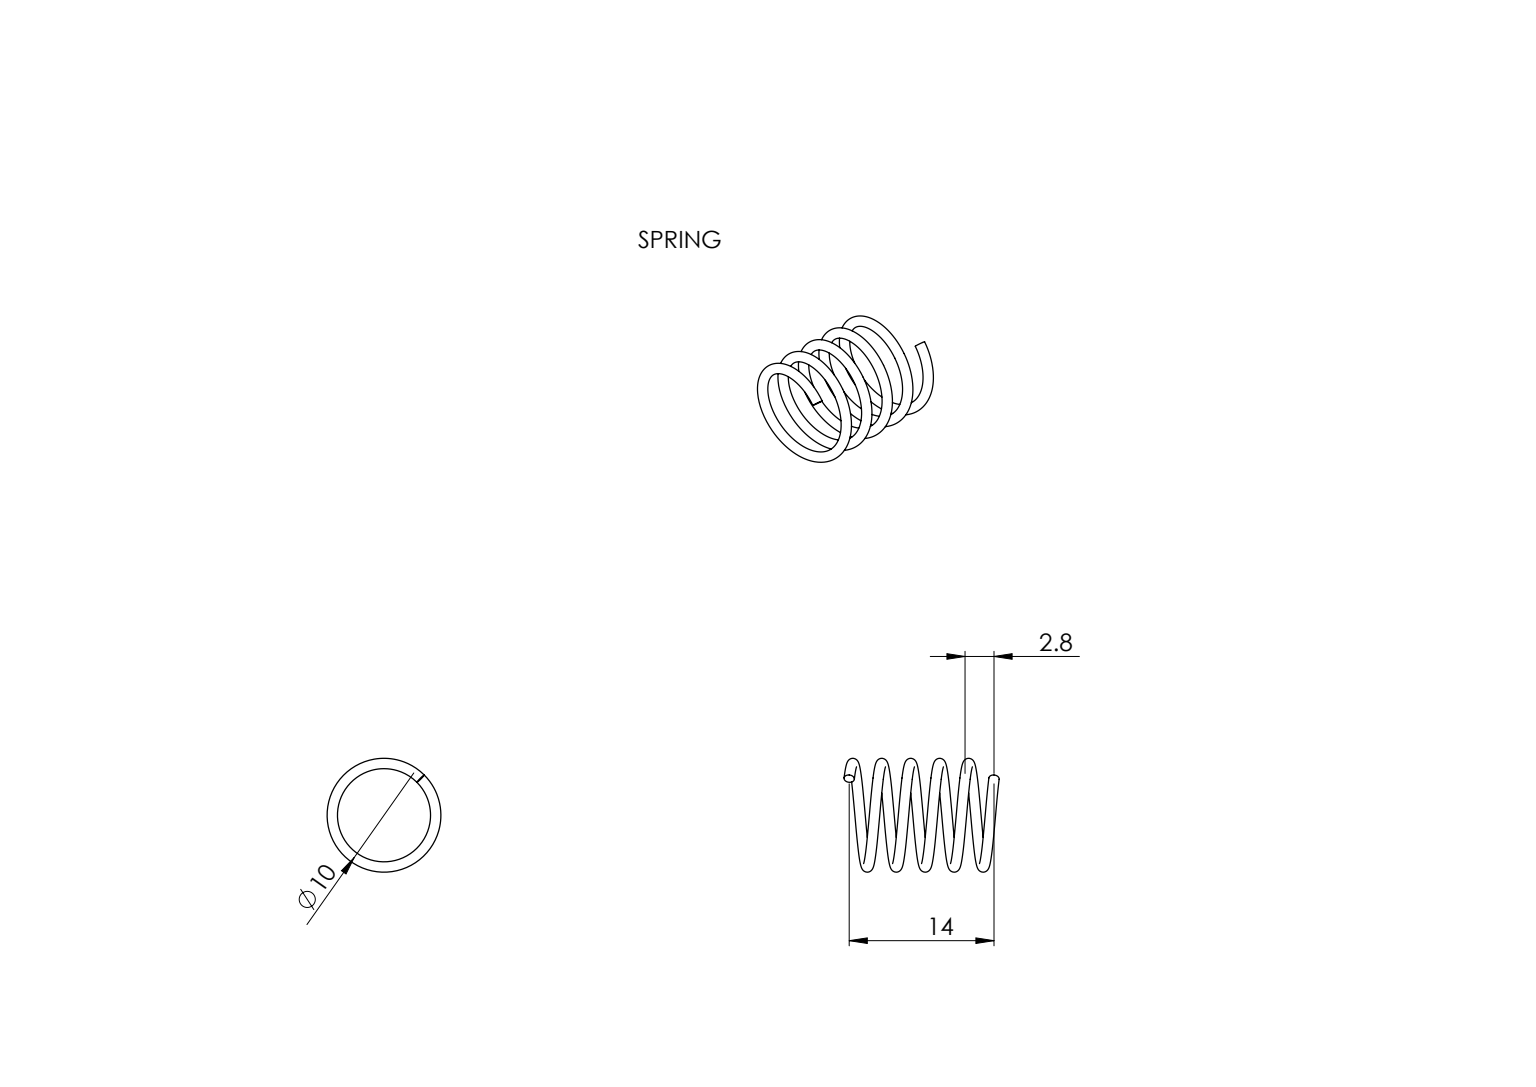
ISO-10303-21;
HEADER;
FILE_DESCRIPTION (('STEP AP214'),
    '1' );
FILE_NAME ('spring.step',
    '2026-10-03T18:28:46',
    ( '' ),
    ( '' ),
    'SwSTEP 2.0',
    'SolidWorks 2026',
    '' );
FILE_SCHEMA (( 'AUTOMOTIVE_DESIGN' ));
ENDSEC;

DATA;
#9=CARTESIAN_POINT ( 'NONE',  ( -2.231261971483764484, -4.173491630687871101, 3.063948283277976081 ) ) ;
#10=ORIENTED_EDGE ( 'NONE', *, *, #5513, .T. ) ;
#14=CARTESIAN_POINT ( 'NONE',  ( 4.089228379062037178, -4.089228379062022967, 0.6999999999999997335 ) ) ;
#18=CARTESIAN_POINT ( 'NONE',  ( 0.9046671180729953798, -5.711843387010016926, 0.9799999999999997602 ) ) ;
#30=CARTESIAN_POINT ( 'NONE',  ( 1.963858260114715870, -4.049832306626327316, 5.443948283277975975 ) ) ;
#40=CARTESIAN_POINT ( 'NONE',  ( 0.7401821875142697849, -4.673326407553650697, 3.779999999999998916 ) ) ;
#43=CARTESIAN_POINT ( 'NONE',  ( -0.9968613283357868893, 5.697241258616382531, 14.57605171672202538 ) ) ;
#49=CARTESIAN_POINT ( 'NONE',  ( 5.432285873273257515, 0.8603895577212793411, 8.679999999999997939 ) ) ;
#51=CARTESIAN_POINT ( 'NONE',  ( -3.889087296526005044, -3.889087296526019255, 1.399999999999999689 ) ) ;
#64=CARTESIAN_POINT ( 'NONE',  ( 3.244753828200538148, 3.119207202478391672, -0.9960517167220231949 ) ) ;
#67=CARTESIAN_POINT ( 'NONE',  ( -0.8603895577212598011, -5.432285873273260179, 6.719999999999999751 ) ) ;
#76=CARTESIAN_POINT ( 'NONE',  ( 4.430710083317573655, 0.7916369971161595354, 1.276051716722023333 ) ) ;
#79=CARTESIAN_POINT ( 'NONE',  ( 4.458484982038663169, 0.6162731882459350219, 2.083948283277976543 ) ) ;
#91=CARTESIAN_POINT ( 'NONE',  ( 4.009529358847659708, -2.042957248827953709, 0.5599999999999999423 ) ) ;
#93=CARTESIAN_POINT ( 'NONE',  ( 4.430710083317573655, 0.7916369971161595354, 6.876051716722023421 ) ) ;
#102=CARTESIAN_POINT ( 'NONE',  ( -3.889087296526005044, -3.889087296526019255, 4.200000000000000178 ) ) ;
#103=CARTESIAN_POINT ( 'NONE',  ( 2.625446233515515537, 5.152728359536502545, 5.459999999999997300 ) ) ;
#104=CARTESIAN_POINT ( 'NONE',  ( -5.697241258616385196, 0.9968613283357647958, 12.02394828327797427 ) ) ;
#117=CARTESIAN_POINT ( 'NONE',  ( 0.7916369971161419938, 4.430710083317576320, 4.323948283277975868 ) ) ;
#120=CARTESIAN_POINT ( 'NONE',  ( 4.089228379062037178, -4.089228379062022967, 9.099999999999999645 ) ) ;
#123=CARTESIAN_POINT ( 'NONE',  ( 0.9046671180729953798, -5.711843387010016926, 9.379999999999997229 ) ) ;
#128=CARTESIAN_POINT ( 'NONE',  ( 3.826313983664925811, 3.951860609387098044, 14.99605171672202175 ) ) ;
#131=CARTESIAN_POINT ( 'NONE',  ( -4.258245684917310925, -2.064922774268914019, 6.143948283277977040 ) ) ;
#134=CARTESIAN_POINT ( 'NONE',  ( -0.9968613283357868893, 5.697241258616382531, 6.176051716722023244 ) ) ;
#139=CARTESIAN_POINT ( 'NONE',  ( 4.215868657802586128, 2.148092372876346801, 5.739999999999998437 ) ) ;
#142=CARTESIAN_POINT ( 'NONE',  ( 3.411736077305382420, -3.279728542977940364, 7.296051716722023350 ) ) ;
#149=CARTESIAN_POINT ( 'NONE',  ( 3.889087296526005488, 3.889087296526018811, 5.599999999999998757 ) ) ;
#151=CARTESIAN_POINT ( 'NONE',  ( 5.432285873273257515, 0.8603895577212793411, 3.079999999999999627 ) ) ;
#152=CARTESIAN_POINT ( 'NONE',  ( -5.152728359536494551, -2.625446233515535077, 1.540000000000000036 ) ) ;
#164=CARTESIAN_POINT ( 'NONE',  ( -4.215868657802586128, -2.148092372876348133, 12.73999999999999488 ) ) ;
#169=CARTESIAN_POINT ( 'NONE',  ( -0.8603895577212598011, -5.432285873273260179, 1.119999999999999885 ) ) ;
#172=CARTESIAN_POINT ( 'NONE',  ( 0.9046671180729953798, -5.711843387010016926, 3.779999999999998916 ) ) ;
#178=CARTESIAN_POINT ( 'NONE',  ( -5.418398423912711870, -0.9480714621563917088, 13.87605171672202253 ) ) ;
#182=CARTESIAN_POINT ( 'NONE',  ( -4.458484982038663169, -0.6162731882459353550, 9.083948283277974767 ) ) ;
#187=CARTESIAN_POINT ( 'NONE',  ( 3.826313983664925811, 3.951860609387098044, 0.9960517167220231949 ) ) ;
#193=CARTESIAN_POINT ( 'NONE',  ( 4.673326407553653361, -0.7401821875142525764, 0.4199999999999999845 ) ) ;
#198=CARTESIAN_POINT ( 'NONE',  ( 4.687928535947288644, -0.6479879772514620662, 4.216051716722023279 ) ) ;
#208=CARTESIAN_POINT ( 'NONE',  ( -4.089228379062038066, 4.089228379062021190, 13.29999999999999538 ) ) ;
#209=CARTESIAN_POINT ( 'NONE',  ( -4.900535883036028828, 2.496947748567499126, 4.759999999999999787 ) ) ;
#210=CARTESIAN_POINT ( 'NONE',  ( -5.711843387010018702, 0.9046671180729746187, 1.819999999999999396 ) ) ;
#223=CARTESIAN_POINT ( 'NONE',  ( -1.963858260114716980, 4.049832306626327316, 1.243948283277976463 ) ) ;
#226=CARTESIAN_POINT ( 'NONE',  ( 2.496947748567516889, -4.900535883036019946, 6.439999999999999503 ) ) ;
#229=CARTESIAN_POINT ( 'NONE',  ( 0.8603895577212593571, 5.432285873273261068, 5.319999999999999396 ) ) ;
#235=CARTESIAN_POINT ( 'NONE',  ( 4.173491630687861331, 2.231261971483781359, 1.136051716722023208 ) ) ;
#237=CARTESIAN_POINT ( 'NONE',  ( -1.963858260114716980, 4.049832306626327316, 4.043948283277976508 ) ) ;
#241=CARTESIAN_POINT ( 'NONE',  ( 4.155232146225751322, -4.023224611898307934, 7.296051716722023350 ) ) ;
#245=CARTESIAN_POINT ( 'NONE',  ( 4.673326407553653361, -0.7401821875142525764, 11.61999999999999922 ) ) ;
#248=CARTESIAN_POINT ( 'NONE',  ( -4.173491630687863108, -2.231261971483782691, 10.93605171672202125 ) ) ;
#257=CARTESIAN_POINT ( 'NONE',  ( 0.7727076532861471003, 5.446173322633805824, 3.516051716722023102 ) ) ;
#258=FACE_OUTER_BOUND ( 'NONE', #8568, .T. ) ;
#259=STYLED_ITEM ( 'NONE', ( #1415 ), #6736 ) ;
#261=CARTESIAN_POINT ( 'NONE',  ( 3.889087296526005488, 3.889087296526018811, 11.19999999999999751 ) ) ;
#273=CARTESIAN_POINT ( 'NONE',  ( -2.231261971483764484, -4.173491630687871101, 5.863948283277976792 ) ) ;
#281=CARTESIAN_POINT ( 'NONE',  ( -2.625446233515515537, -5.152728359536502545, 9.659999999999996589 ) ) ;
#286=CARTESIAN_POINT ( 'NONE',  ( -4.687928535947287756, 0.6479879772514611780, 8.416051716722021681 ) ) ;
#290=CARTESIAN_POINT ( 'NONE',  ( -4.860232935257354114, 2.576046737280751842, 0.9639482832779766586 ) ) ;
#293=CARTESIAN_POINT ( 'NONE',  ( -0.7727076532861475444, -5.446173322633804048, 7.716051716722023279 ) ) ;
#298=CARTESIAN_POINT ( 'NONE',  ( -2.148092372876330813, -4.215868657802594122, 6.859999999999999432 ) ) ;
#300=CARTESIAN_POINT ( 'NONE',  ( -4.173491630687863108, -2.231261971483782691, 8.136051716722024096 ) ) ;
#308=CARTESIAN_POINT ( 'NONE',  ( 5.432285873273257515, 0.8603895577212793411, 11.47999999999999865 ) ) ;
#309=CARTESIAN_POINT ( 'NONE',  ( 3.889087296526005488, 3.889087296526018811, 2.799999999999999378 ) ) ;
#310=CARTESIAN_POINT ( 'NONE',  ( 4.089228379062037178, -4.089228379062022967, 11.90000000000000036 ) ) ;
#321=CARTESIAN_POINT ( 'NONE',  ( 3.969226411068985882, -2.122056237541205981, 10.76394828327797626 ) ) ;
#325=CARTESIAN_POINT ( 'NONE',  ( -2.625446233515515981, -5.152728359536500768, 12.45999999999999552 ) ) ;
#327=CARTESIAN_POINT ( 'NONE',  ( -2.496947748567517333, 4.900535883036019058, 7.839999999999999858 ) ) ;
#332=CARTESIAN_POINT ( 'NONE',  ( 0.6162731882459174804, 4.458484982038668498, 11.91605171672202346 ) ) ;
#335=CARTESIAN_POINT ( 'NONE',  ( 0.8124729078102063129, -5.726445515403652209, -0.01605171672202330979 ) ) ;
#342=CARTESIAN_POINT ( 'NONE',  ( 3.889087296526005488, 3.889087296526018811, 13.99999999999999822 ) ) ;
#348=CARTESIAN_POINT ( 'NONE',  ( 2.042957248827968808, -4.009529358847652603, 6.439999999999999503 ) ) ;
#350=CARTESIAN_POINT ( 'NONE',  ( -4.009529358847660596, 2.042957248827953265, 1.959999999999999964 ) ) ;
#360=CARTESIAN_POINT ( 'NONE',  ( -0.7727076532861475444, -5.446173322633804048, 2.116051716722023190 ) ) ;
#361=CARTESIAN_POINT ( 'NONE',  ( -0.8603895577212598011, -5.432285873273260179, 12.31999999999999851 ) ) ;
#363=CARTESIAN_POINT ( 'NONE',  ( -5.152728359536494551, -2.625446233515535077, 7.139999999999997016 ) ) ;
#375=CARTESIAN_POINT ( 'NONE',  ( 3.279728542977952799, -3.411736077305369541, 10.90394828327797327 ) ) ;
#378=CARTESIAN_POINT ( 'NONE',  ( 2.496947748567516889, -4.900535883036019946, 12.03999999999999915 ) ) ;
#385=CARTESIAN_POINT ( 'NONE',  ( -4.430710083317573655, -0.7916369971161599794, 11.07605171672202182 ) ) ;
#388=CARTESIAN_POINT ( 'NONE',  ( -5.446173322633801384, -0.7727076532861678615, 0.6839482832779766319 ) ) ;
#396=CARTESIAN_POINT ( 'NONE',  ( -0.7039550926810301812, -4.444597532678121965, 12.31999999999999851 ) ) ;
#400=CARTESIAN_POINT ( 'NONE',  ( -4.173491630687863108, -2.231261971483782691, 13.73605171672202019 ) ) ;
#410=CARTESIAN_POINT ( 'NONE',  ( -3.826313983664925811, -3.951860609387098489, 2.396051716722022551 ) ) ;
#411=CARTESIAN_POINT ( 'NONE',  ( 2.625446233515515537, 5.152728359536502545, 11.05999999999999872 ) ) ;
#412=CARTESIAN_POINT ( 'NONE',  ( -0.9046671180729963790, 5.711843387010016926, 7.979999999999999538 ) ) ;
#420=CARTESIAN_POINT ( 'NONE',  ( 3.535533905932731980, 3.535533905932744414, 13.99999999999999822 ) ) ;
#425=CARTESIAN_POINT ( 'NONE',  ( 1.963858260114715870, -4.049832306626327316, 11.04394828327797562 ) ) ;
#438=CARTESIAN_POINT ( 'NONE',  ( 3.411736077305382420, -3.279728542977940364, 12.89605171672202211 ) ) ;
#440=CARTESIAN_POINT ( 'NONE',  ( -5.697241258616385196, 0.9968613283357647958, 0.8239482832779764232 ) ) ;
#450=CARTESIAN_POINT ( 'NONE',  ( -2.148092372876330813, -4.215868657802594122, 9.659999999999996589 ) ) ;
#451=CARTESIAN_POINT ( 'NONE',  ( -0.7039550926810301812, -4.444597532678121965, 6.719999999999999751 ) ) ;
#460=CARTESIAN_POINT ( 'NONE',  ( 2.542276634908080535, 5.195105386651229118, 9.256051716722023315 ) ) ;
#461=CARTESIAN_POINT ( 'NONE',  ( -0.8603895577212598011, -5.432285873273260179, 9.519999999999999574 ) ) ;
#462=CARTESIAN_POINT ( 'NONE',  ( 5.152728359536493663, 2.625446233515533745, 11.33999999999999808 ) ) ;
#475=CARTESIAN_POINT ( 'NONE',  ( -0.7916369971161423269, -4.430710083317576320, 11.32394828327797676 ) ) ;
#478=CARTESIAN_POINT ( 'NONE',  ( -3.889087296526005044, -3.889087296526019255, 9.799999999999998934 ) ) ;
#486=CARTESIAN_POINT ( 'NONE',  ( -3.345732310141667831, 3.345732310141653620, 2.099999999999999201 ) ) ;
#488=CARTESIAN_POINT ( 'NONE',  ( -0.9480714621563718358, -5.418398423912716311, 0.1239482832779766203 ) ) ;
#498=CARTESIAN_POINT ( 'NONE',  ( 0.7401821875142697849, -4.673326407553650697, 3.779999999999998472 ) ) ;
#506=CARTESIAN_POINT ( 'NONE',  ( 0.7727076532861471003, 5.446173322633805824, 6.316051716722022924 ) ) ;
#513=FILL_AREA_STYLE ('',( #1309 ) ) ;
#524=CARTESIAN_POINT ( 'NONE',  ( 2.417848759854264618, -4.940838830814695548, 5.443948283277975975 ) ) ;
#539=CARTESIAN_POINT ( 'NONE',  ( -2.122056237541221968, 3.969226411068977889, 11.63605171672202232 ) ) ;
#542=CARTESIAN_POINT ( 'NONE',  ( -0.9480714621563718358, -5.418398423912716311, 11.32394828327797676 ) ) ;
#553=CARTESIAN_POINT ( 'NONE',  ( -3.411736077305382420, 3.279728542977939476, 14.29605171672202424 ) ) ;
#561=CARTESIAN_POINT ( 'NONE',  ( 5.726445515403654873, -0.8124729078101852187, 12.61605171672202097 ) ) ;
#575=CARTESIAN_POINT ( 'NONE',  ( -0.9480714621563718358, -5.418398423912716311, 0.1239482832779766203 ) ) ;
#587=CARTESIAN_POINT ( 'NONE',  ( -3.181980515339458027, -3.181980515339470905, 6.999999999999999112 ) ) ;
#590=CARTESIAN_POINT ( 'NONE',  ( -0.8124729078102072011, 5.726445515403652209, 12.58394828327797477 ) ) ;
#605=CARTESIAN_POINT ( 'NONE',  ( 0.7039550926810297371, 4.444597532678122853, 8.119999999999999218 ) ) ;
#615=CARTESIAN_POINT ( 'NONE',  ( -5.110351332421769754, -2.708615832122969191, 10.93605171672202125 ) ) ;
#620=CARTESIAN_POINT ( 'NONE',  ( -0.7727076532861475444, -5.446173322633804048, 10.51605171672202133 ) ) ;
#629=CARTESIAN_POINT ( 'NONE',  ( 0.9480714621563713917, 5.418398423912717199, 7.123948283277974802 ) ) ;
#638=CARTESIAN_POINT ( 'NONE',  ( 4.215868657802586128, 2.148092372876346801, 2.939999999999999059 ) ) ;
#640=CARTESIAN_POINT ( 'NONE',  ( 2.708615832122949652, 5.110351332421781301, 12.86394828327797768 ) ) ;
#642=ADVANCED_FACE ( 'NONE', ( #9719 ), #6462, .T. ) ;
#653=CARTESIAN_POINT ( 'NONE',  ( -4.009529358847660596, 2.042957248827953265, 13.15999999999999837 ) ) ;
#663=CARTESIAN_POINT ( 'NONE',  ( -2.576046737280769605, 4.860232935257343456, 11.63605171672202232 ) ) ;
#670=CARTESIAN_POINT ( 'NONE',  ( 4.687928535947288644, -0.6479879772514620662, 1.416051716722023235 ) ) ;
#674=SURFACE_STYLE_FILL_AREA ( #513 ) ;
#682=CARTESIAN_POINT ( 'NONE',  ( -2.417848759854264618, 4.940838830814694660, 4.043948283277976508 ) ) ;
#699=CARTESIAN_POINT ( 'NONE',  ( -4.215868657802586128, -2.148092372876348133, 7.139999999999997016 ) ) ;
#702=CARTESIAN_POINT ( 'NONE',  ( 3.951860609387084722, 3.826313983664940022, 7.403948283277976827 ) ) ;
#706=CARTESIAN_POINT ( 'NONE',  ( -2.625446233515515537, -5.152728359536502545, 1.259999999999999787 ) ) ;
#715=CARTESIAN_POINT ( 'NONE',  ( -4.215868657802586128, -2.148092372876348133, 12.73999999999999488 ) ) ;
#726=CARTESIAN_POINT ( 'NONE',  ( -4.430710083317573655, -0.7916369971161599794, 2.676051716722023244 ) ) ;
#735=CARTESIAN_POINT ( 'NONE',  ( 0.9046671180729951578, -5.711843387010016926, 6.579999999999999183 ) ) ;
#738=CARTESIAN_POINT ( 'NONE',  ( -4.860232935257354114, 2.576046737280751842, 0.9639482832779766586 ) ) ;
#751=CARTESIAN_POINT ( 'NONE',  ( 4.009529358847659708, -2.042957248827953709, 3.359999999999999876 ) ) ;
#754=CARTESIAN_POINT ( 'NONE',  ( -5.195105386651219348, -2.542276634908102295, 8.943948283277975975 ) ) ;
#755=AXIS2_PLACEMENT_3D ( 'NONE', #9759, #8791, #4917 ) ;
#767=CARTESIAN_POINT ( 'NONE',  ( 1.963858260114715870, -4.049832306626327316, -0.1560517167220233370 ) ) ;
#780=CARTESIAN_POINT ( 'NONE',  ( 2.064922774268895811, 4.258245684917319807, 3.656051716722022782 ) ) ;
#790=CARTESIAN_POINT ( 'NONE',  ( 4.900535883036028828, -2.496947748567499126, 8.959999999999999076 ) ) ;
#792=CARTESIAN_POINT ( 'NONE',  ( 4.023224611898322145, -4.155232146225737111, 10.90394828327797327 ) ) ;
#804=CARTESIAN_POINT ( 'NONE',  ( 4.258245684917310037, 2.064922774268912686, 1.943948283277976419 ) ) ;
#807=CARTESIAN_POINT ( 'NONE',  ( 2.496947748567516889, -4.900535883036019946, 3.639999999999999680 ) ) ;
#810=CARTESIAN_POINT ( 'NONE',  ( 0.8603895577212593571, 5.432285873273261068, 2.519999999999999574 ) ) ;
#817=CARTESIAN_POINT ( 'NONE',  ( -0.7916369971161423269, -4.430710083317576320, 0.1239482832779766203 ) ) ;
#825=CARTESIAN_POINT ( 'NONE',  ( 4.009529358847659708, -2.042957248827953709, 3.359999999999999876 ) ) ;
#830=CARTESIAN_POINT ( 'NONE',  ( -0.9968613283357868893, 5.697241258616382531, 11.77605171672202289 ) ) ;
#839=CARTESIAN_POINT ( 'NONE',  ( -4.089228379062038066, 4.089228379062021190, 7.699999999999998401 ) ) ;
#841=CARTESIAN_POINT ( 'NONE',  ( 2.417848759854264618, -4.940838830814695548, 11.04394828327797562 ) ) ;
#855=CARTESIAN_POINT ( 'NONE',  ( 3.969226411068985882, -2.122056237541205981, 5.163948283277975726 ) ) ;
#861=CARTESIAN_POINT ( 'NONE',  ( 5.711843387010018702, -0.9046671180729751738, 8.820000000000000284 ) ) ;
#873=CARTESIAN_POINT ( 'NONE',  ( 4.430710083317573655, 0.7916369971161595354, 6.876051716722023421 ) ) ;
#877=CARTESIAN_POINT ( 'NONE',  ( -3.969226411068985882, 2.122056237541205537, 6.563948283277975193 ) ) ;
#889=CARTESIAN_POINT ( 'NONE',  ( -3.411736077305382420, 3.279728542977939476, 8.696051716722022817 ) ) ;
#894=CARTESIAN_POINT ( 'NONE',  ( -2.625446233515515981, -5.152728359536500768, 4.059999999999999609 ) ) ;
#896=CARTESIAN_POINT ( 'NONE',  ( -3.951860609387083834, -3.826313983664940466, 11.60394828327797434 ) ) ;
#908=CARTESIAN_POINT ( 'NONE',  ( 2.231261971483764484, 4.173491630687871101, 4.463948283277976437 ) ) ;
#911=CARTESIAN_POINT ( 'NONE',  ( -5.711843387010018702, 0.9046671180729746187, 1.819999999999999396 ) ) ;
#914=CARTESIAN_POINT ( 'NONE',  ( -5.152728359536494551, -2.625446233515535521, 4.339999999999999858 ) ) ;
#919=CARTESIAN_POINT ( 'NONE',  ( 0.8323763977770604061, -4.658724279160015413, 1.976051716722022844 ) ) ;
#922=CARTESIAN_POINT ( 'NONE',  ( -3.244753828200538148, -3.119207202478392116, 3.203948283277977094 ) ) ;
#933=CARTESIAN_POINT ( 'NONE',  ( 4.673326407553653361, -0.7401821875142525764, 3.219999999999999751 ) ) ;
#937=CARTESIAN_POINT ( 'NONE',  ( -3.411736077305382420, 3.279728542977939476, 5.896051716722023883 ) ) ;
#947=CARTESIAN_POINT ( 'NONE',  ( 0.9046671180729951578, -5.711843387010016926, 3.779999999999998472 ) ) ;
#948=CARTESIAN_POINT ( 'NONE',  ( 4.900535883036028828, -2.496947748567499126, 6.159999999999999254 ) ) ;
#949=CARTESIAN_POINT ( 'NONE',  ( -2.496947748567517333, 4.900535883036019058, 2.239999999999999769 ) ) ;
#961=CARTESIAN_POINT ( 'NONE',  ( 3.244753828200538148, 3.119207202478391672, 4.603948283277976117 ) ) ;
#964=CARTESIAN_POINT ( 'NONE',  ( 4.900535883036028828, -2.496947748567499126, 6.159999999999999254 ) ) ;
#967=CARTESIAN_POINT ( 'NONE',  ( -4.089228379062038066, 4.089228379062022078, 4.899999999999999467 ) ) ;
#971=CARTESIAN_POINT ( 'NONE',  ( 4.687928535947288644, -0.6479879772514620662, 7.016051716722022213 ) ) ;
#974=CARTESIAN_POINT ( 'NONE',  ( -3.969226411068985882, 2.122056237541205537, 0.9639482832779766586 ) ) ;
#977=CARTESIAN_POINT ( 'NONE',  ( 4.155232146225751322, -4.023224611898307934, 1.696051716722023484 ) ) ;
#984=EDGE_CURVE ( 'NONE', #5388, #5138, #5355, .T. ) ;
#986=CARTESIAN_POINT ( 'NONE',  ( 3.411736077305382420, -3.279728542977940364, 12.89605171672202211 ) ) ;
#992=CARTESIAN_POINT ( 'NONE',  ( -5.418398423912711870, -0.9480714621563917088, 2.676051716722023244 ) ) ;
#993=CARTESIAN_POINT ( 'NONE',  ( 4.089228379062037178, -4.089228379062022967, 3.499999999999998668 ) ) ;
#994=CARTESIAN_POINT ( 'NONE',  ( -5.432285873273256627, -0.8603895577212797852, 4.479999999999999538 ) ) ;
#1007=CARTESIAN_POINT ( 'NONE',  ( 0.6479879772514793856, -4.687928535947285091, 2.783948283277976277 ) ) ;
#1011=CARTESIAN_POINT ( 'NONE',  ( 2.496947748567516889, -4.900535883036019946, 0.8399999999999999689 ) ) ;
#1013=CARTESIAN_POINT ( 'NONE',  ( -3.889087296526005044, -3.889087296526019255, 9.799999999999998934 ) ) ;
#1019=CARTESIAN_POINT ( 'NONE',  ( -2.122056237541221968, 3.969226411068977889, 6.036051716722022675 ) ) ;
#1021=CARTESIAN_POINT ( 'NONE',  ( -2.231261971483764484, -4.173491630687871101, 5.863948283277976792 ) ) ;
#1028=CARTESIAN_POINT ( 'NONE',  ( 5.726445515403654873, -0.8124729078101852187, 1.416051716722023235 ) ) ;
#1040=CARTESIAN_POINT ( 'NONE',  ( 4.430710083317573655, 0.7916369971161595354, 9.676051716722021467 ) ) ;
#1050=CARTESIAN_POINT ( 'NONE',  ( -0.9968613283357868893, 5.697241258616382531, 3.376051716722022977 ) ) ;
#1051=CARTESIAN_POINT ( 'NONE',  ( 2.625446233515515537, 5.152728359536502545, 8.259999999999999787 ) ) ;
#1052=CARTESIAN_POINT ( 'NONE',  ( -3.889087296526005044, -3.889087296526019255, 12.59999999999999787 ) ) ;
#1062=PLANE ( 'NONE',  #4221 ) ;
#1064=CARTESIAN_POINT ( 'NONE',  ( -4.258245684917310925, -2.064922774268914019, 11.74394828327797846 ) ) ;
#1070=CARTESIAN_POINT ( 'NONE',  ( -4.900535883036028828, 2.496947748567499126, 7.559999999999998721 ) ) ;
#1075=CARTESIAN_POINT ( 'NONE',  ( -0.9968613283357868893, 5.697241258616382531, 14.57605171672202538 ) ) ;
#1077=CARTESIAN_POINT ( 'NONE',  ( -4.023224611898323033, 4.155232146225737111, 1.103948283277976561 ) ) ;
#1081=CARTESIAN_POINT ( 'NONE',  ( 5.726445515403654873, -0.8124729078101852187, 4.216051716722023279 ) ) ;
#1086=CARTESIAN_POINT ( 'NONE',  ( -4.444597532678119300, -0.7039550926810477227, 7.279999999999999361 ) ) ;
#1087=CARTESIAN_POINT ( 'NONE',  ( 3.411736077305382420, -3.279728542977940364, 4.496051716722022640 ) ) ;
#1088=( BOUNDED_CURVE ( )  B_SPLINE_CURVE ( 2, ( #8758, #1499, #6470, #3992, #9727, #9676, #2406, #18, #4720, #706, #5623, #7162, #10419, #2346, #5569, #1559, #8817, #1609, #810, #4040, #7271, #2458, #5673, #10042, #9126, #1816, #4141, #172, #5877, #9183, #6631, #914, #7489, #1867, #7427, #967, #4193, #8342, #229, #1920, #6783, #3406, #1714, #9883, #3556, #5092, #2763, #7583, #2561, #9081, #2613, #1122, #5144, #5828, #1070, #4344, #327, #5929, #5978, #1763, #4940, #5040, #3505, #9830, #8182, #8238, #8287, #123, #4243, #281, #1013, #7536, #6722, #6574, #8391, #4293, #3456, #6677, #7379, #9026, #3348, #5776, #9935, #2661, #9985, #2710, #4990, #2075, #10194, #2021, #2973, #7644, #2921, #3022, #9447, #2176, #10293, #9235, #1167, #4395, #4550 ),
 .UNSPECIFIED., .F., .T. ) 
 B_SPLINE_CURVE_WITH_KNOTS ( ( 3, 2, 2, 2, 2, 2, 2, 2, 2, 2, 2, 2, 2, 2, 2, 2, 2, 2, 2, 2, 2, 2, 2, 2, 2, 2, 2, 2, 2, 2, 2, 2, 2, 2, 2, 2, 2, 2, 2, 2, 2, 2, 2, 2, 2, 2, 2, 2, 2, 2, 3 ),
 ( 0.000000000000000000, 0.02000000000000000042, 0.04000000000000000083, 0.05999999999999999778, 0.08000000000000000167, 0.1000000000000000056, 0.1199999999999999956, 0.1400000000000000133, 0.1600000000000000033, 0.1799999999999999933, 0.2000000000000000111, 0.2200000000000000011, 0.2399999999999999911, 0.2600000000000000089, 0.2800000000000000266, 0.2999999999999999889, 0.3200000000000000067, 0.3400000000000000244, 0.3599999999999999867, 0.3800000000000000044, 0.4000000000000000222, 0.4199999999999999845, 0.4400000000000000022, 0.4600000000000000200, 0.4799999999999999822, 0.5000000000000000000, 0.5200000000000000178, 0.5400000000000000355, 0.5600000000000000533, 0.5799999999999999600, 0.5999999999999999778, 0.6199999999999999956, 0.6400000000000000133, 0.6600000000000000311, 0.6800000000000000488, 0.6999999999999999556, 0.7199999999999999734, 0.7399999999999999911, 0.7600000000000000089, 0.7800000000000000266, 0.8000000000000000444, 0.8199999999999999512, 0.8399999999999999689, 0.8599999999999999867, 0.8800000000000000044, 0.9000000000000000222, 0.9200000000000000400, 0.9399999999999999467, 0.9599999999999999645, 0.9799999999999999822, 1.000000000000000000 ),
 .UNSPECIFIED. ) 
 CURVE ( )  GEOMETRIC_REPRESENTATION_ITEM ( )  RATIONAL_B_SPLINE_CURVE ( ( 1.000000000000000000, 0.9510565162951535312, 1.000000000000000000, 0.9510565162951535312, 1.000000000000000000, 0.9510565162951535312, 1.000000000000000000, 0.9510565162951535312, 1.000000000000000000, 0.9510565162951535312, 1.000000000000000000, 0.9510565162951535312, 1.000000000000000000, 0.9510565162951535312, 1.000000000000000000, 0.9510565162951535312, 1.000000000000000000, 0.9510565162951535312, 1.000000000000000000, 0.9510565162951535312, 1.000000000000000000, 0.9510565162951535312, 1.000000000000000000, 0.9510565162951535312, 1.000000000000000000, 0.9510565162951535312, 1.000000000000000000, 0.9510565162951535312, 1.000000000000000000, 0.9510565162951535312, 1.000000000000000000, 0.9510565162951535312, 1.000000000000000000, 0.9510565162951535312, 1.000000000000000000, 0.9510565162951535312, 1.000000000000000000, 0.9510565162951535312, 1.000000000000000000, 0.9510565162951535312, 1.000000000000000000, 0.9510565162951535312, 1.000000000000000000, 0.9510565162951535312, 1.000000000000000000, 0.9510565162951535312, 1.000000000000000000, 0.9510565162951535312, 1.000000000000000000, 0.9510565162951535312, 1.000000000000000000, 0.9510565162951535312, 1.000000000000000000, 0.9510565162951535312, 1.000000000000000000, 0.9510565162951535312, 1.000000000000000000, 0.9510565162951535312, 1.000000000000000000, 0.9510565162951535312, 1.000000000000000000, 0.9510565162951535312, 1.000000000000000000, 0.9510565162951535312, 1.000000000000000000, 0.9510565162951535312, 1.000000000000000000, 0.9510565162951535312, 1.000000000000000000, 0.9510565162951535312, 1.000000000000000000, 0.9510565162951535312, 1.000000000000000000, 0.9510565162951535312, 1.000000000000000000, 0.9510565162951535312, 1.000000000000000000, 0.9510565162951535312, 1.000000000000000000, 0.9510565162951535312, 1.000000000000000000, 0.9510565162951535312, 1.000000000000000000, 0.9510565162951535312, 1.000000000000000000, 0.9510565162951535312, 1.000000000000000000, 0.9510565162951535312, 1.000000000000000000, 0.9510565162951535312, 1.000000000000000000, 0.9510565162951535312, 1.000000000000000000, 0.9510565162951535312, 1.000000000000000000, 0.9510565162951535312, 1.000000000000000000, 0.9510565162951535312, 1.000000000000000000, 0.9510565162951535312, 1.000000000000000000 ) ) 
 REPRESENTATION_ITEM ( '' )  );
#1097=CARTESIAN_POINT ( 'NONE',  ( 5.152728359536493663, 2.625446233515533745, 11.33999999999999808 ) ) ;
#1098=CARTESIAN_POINT ( 'NONE',  ( -5.432285873273256627, -0.8603895577212797852, 1.679999999999999938 ) ) ;
#1099=CARTESIAN_POINT ( 'NONE',  ( 0.9046671180729951578, -5.711843387010016926, 9.379999999999995453 ) ) ;
#1110=AXIS2_PLACEMENT_3D ( 'NONE', #9054, #3327, #4117 ) ;
#1113=CARTESIAN_POINT ( 'NONE',  ( 0.6479879772514793856, -4.687928535947285091, 11.18394828327797441 ) ) ;
#1119=CARTESIAN_POINT ( 'NONE',  ( -4.900535883036028828, 2.496947748567499126, 10.35999999999999943 ) ) ;
#1122=CARTESIAN_POINT ( 'NONE',  ( -5.152728359536494551, -2.625446233515535521, 7.139999999999998792 ) ) ;
#1127=CARTESIAN_POINT ( 'NONE',  ( -4.444597532678119300, -0.7039550926810477227, 1.679999999999999938 ) ) ;
#1130=CARTESIAN_POINT ( 'NONE',  ( 0.9480714621563713917, 5.418398423912717199, 1.523948283277976268 ) ) ;
#1133=CARTESIAN_POINT ( 'NONE',  ( -5.726445515403654873, 0.8124729078101847746, 8.416051716722021681 ) ) ;
#1137=CARTESIAN_POINT ( 'NONE',  ( -3.181980515339458027, -3.181980515339470905, 6.999999999999999112 ) ) ;
#1139=CARTESIAN_POINT ( 'NONE',  ( 3.345732310141667387, -3.345732310141653620, 0.6999999999999997335 ) ) ;
#1147=CARTESIAN_POINT ( 'NONE',  ( 0.8603895577212593571, 5.432285873273261068, 13.71999999999999886 ) ) ;
#1148=CARTESIAN_POINT ( 'NONE',  ( -3.889087296526005044, -3.889087296526019255, 9.799999999999998934 ) ) ;
#1149=CARTESIAN_POINT ( 'NONE',  ( -4.900535883036028828, 2.496947748567499126, 13.15999999999999837 ) ) ;
#1161=CARTESIAN_POINT ( 'NONE',  ( -0.7916369971161423269, -4.430710083317576320, 5.723948283277976223 ) ) ;
#1165=CARTESIAN_POINT ( 'NONE',  ( 4.089228379062037178, -4.089228379062022967, 11.90000000000000036 ) ) ;
#1167=CARTESIAN_POINT ( 'NONE',  ( 0.8603895577212593571, 5.432285873273261068, 13.71999999999999886 ) ) ;
#1169=EDGE_CURVE ( 'NONE', #5388, #2194, #3876, .T. ) ;
#1174=CARTESIAN_POINT ( 'NONE',  ( -4.173491630687863108, -2.231261971483782691, 10.93605171672202125 ) ) ;
#1177=CARTESIAN_POINT ( 'NONE',  ( -3.951860609387083834, -3.826313983664940466, 3.203948283277977094 ) ) ;
#1179=CIRCLE ( 'NONE', #7790, 0.5000000000000000000 ) ;
#1182=CARTESIAN_POINT ( 'NONE',  ( -2.576046737280769605, 4.860232935257343456, 6.036051716722022675 ) ) ;
#1187=( GEOMETRIC_REPRESENTATION_CONTEXT ( 3 ) GLOBAL_UNCERTAINTY_ASSIGNED_CONTEXT ( ( #1667 ) ) GLOBAL_UNIT_ASSIGNED_CONTEXT ( ( #10273, #1625, #3157 ) ) REPRESENTATION_CONTEXT ( 'NONE', 'WORKASPACE' ) );
#1188=CARTESIAN_POINT ( 'NONE',  ( 0.7039550926810297371, 4.444597532678122853, 10.91999999999999993 ) ) ;
#1191=CARTESIAN_POINT ( 'NONE',  ( -0.8323763977770610722, 4.658724279160015413, 14.57605171672202538 ) ) ;
#1203=CARTESIAN_POINT ( 'NONE',  ( -5.152728359536494551, -2.625446233515535077, 12.73999999999999488 ) ) ;
#1204=CARTESIAN_POINT ( 'NONE',  ( 5.711843387010018702, -0.9046671180729751738, 11.61999999999999922 ) ) ;
#1206=CARTESIAN_POINT ( 'NONE',  ( 2.625446233515515537, 5.152728359536502545, 8.259999999999999787 ) ) ;
#1218=CARTESIAN_POINT ( 'NONE',  ( -2.231261971483764484, -4.173491630687871101, 8.663948283277974838 ) ) ;
#1228=CARTESIAN_POINT ( 'NONE',  ( 2.064922774268895811, 4.258245684917319807, 14.85605171672202296 ) ) ;
#1230=CARTESIAN_POINT ( 'NONE',  ( 0.7916369971161419938, 4.430710083317576320, 9.923948283277976401 ) ) ;
#1241=CARTESIAN_POINT ( 'NONE',  ( -4.444597532678119300, -0.7039550926810477227, 12.87999999999999901 ) ) ;
#1244=CARTESIAN_POINT ( 'NONE',  ( 3.345732310141667387, -3.345732310141653620, 6.299999999999999822 ) ) ;
#1254=CARTESIAN_POINT ( 'NONE',  ( -4.155232146225753098, 4.023224611898306158, 8.696051716722022817 ) ) ;
#1255=CARTESIAN_POINT ( 'NONE',  ( -4.089228379062038066, 4.089228379062021190, 10.50000000000000000 ) ) ;
#1256=CARTESIAN_POINT ( 'NONE',  ( -4.089228379062038066, 4.089228379062021190, 4.900000000000000355 ) ) ;
#1268=CARTESIAN_POINT ( 'NONE',  ( -0.7916369971161423269, -4.430710083317576320, 8.523948283277976046 ) ) ;
#1281=CARTESIAN_POINT ( 'NONE',  ( -0.6162731882459178134, -4.458484982038665834, 10.51605171672202133 ) ) ;
#1283=CARTESIAN_POINT ( 'NONE',  ( -3.279728542977953687, 3.411736077305369541, 12.30394828327797718 ) ) ;
#1291=ORIENTED_EDGE ( 'NONE', *, *, #984, .F. ) ;
#1295=CARTESIAN_POINT ( 'NONE',  ( -0.7401821875142701179, 4.673326407553649808, 2.379999999999999893 ) ) ;
#1303=CARTESIAN_POINT ( 'NONE',  ( -0.7727076532861475444, -5.446173322633804048, 7.716051716722023279 ) ) ;
#1309=FILL_AREA_STYLE_COLOUR ( '', #10249 ) ;
#1317=CARTESIAN_POINT ( 'NONE',  ( 5.446173322633801384, 0.7727076532861675284, 7.683948283277975300 ) ) ;
#1327=CARTESIAN_POINT ( 'NONE',  ( 4.173491630687861331, 2.231261971483781359, 9.536051716722020899 ) ) ;
#1329=CARTESIAN_POINT ( 'NONE',  ( 5.195105386651219348, 2.542276634908100075, 10.34394828327797633 ) ) ;
#1344=CARTESIAN_POINT ( 'NONE',  ( -0.6162731882459178134, -4.458484982038665834, 13.31605171672202204 ) ) ;
#1355=CARTESIAN_POINT ( 'NONE',  ( 4.940838830814703542, -2.417848759854246410, 9.956051716722022604 ) ) ;
#1371=CARTESIAN_POINT ( 'NONE',  ( -4.023224611898323033, 4.155232146225737111, 6.703948283277976650 ) ) ;
#1385=CARTESIAN_POINT ( 'NONE',  ( 0.7401821875142697849, -4.673326407553650697, 6.579999999999999183 ) ) ;
#1387=CARTESIAN_POINT ( 'NONE',  ( -2.708615832122950096, -5.110351332421780413, 5.863948283277976792 ) ) ;
#1399=CARTESIAN_POINT ( 'NONE',  ( 0.7401821875142697849, -4.673326407553650697, 12.17999999999999439 ) ) ;
#1407=CARTESIAN_POINT ( 'NONE',  ( 0.9968613283357860011, -5.697241258616382531, 13.17605171672201969 ) ) ;
#1412=CARTESIAN_POINT ( 'NONE',  ( 4.173491630687861331, 2.231261971483781359, 1.136051716722023208 ) ) ;
#1415=PRESENTATION_STYLE_ASSIGNMENT (( #5383 ) ) ;
#1422=CARTESIAN_POINT ( 'NONE',  ( 5.446173322633801384, 0.7727076532861675284, 4.883948283277976365 ) ) ;
#1435=CARTESIAN_POINT ( 'NONE',  ( -3.181980515339458027, -3.181980515339470905, 9.799999999999998934 ) ) ;
#1439=CARTESIAN_POINT ( 'NONE',  ( -5.195105386651219348, -2.542276634908102295, 11.74394828327797846 ) ) ;
#1443=PRODUCT_CONTEXT ( 'NONE', #5988, 'mechanical' ) ;
#1454=CARTESIAN_POINT ( 'NONE',  ( 0.7039550926810297371, 4.444597532678122853, 13.71999999999999886 ) ) ;
#1464=CARTESIAN_POINT ( 'NONE',  ( 5.418398423912711870, 0.9480714621563913758, 6.876051716722023421 ) ) ;
#1469=CARTESIAN_POINT ( 'NONE',  ( 4.940838830814703542, -2.417848759854246410, 9.956051716722022604 ) ) ;
#1477=CARTESIAN_POINT ( 'NONE',  ( -5.446173322633801384, -0.7727076532861678615, 0.6839482832779766319 ) ) ;
#1491=CARTESIAN_POINT ( 'NONE',  ( 3.181980515339458471, 3.181980515339470461, 11.19999999999999751 ) ) ;
#1494=CARTESIAN_POINT ( 'NONE',  ( 0.9480714621563713917, 5.418398423912717199, 7.123948283277974802 ) ) ;
#1499=CARTESIAN_POINT ( 'NONE',  ( 5.152728359536493663, 2.625446233515533745, 0.1399999999999999578 ) ) ;
#1508=CARTESIAN_POINT ( 'NONE',  ( -4.673326407553653361, 0.7401821875142517992, 7.419999999999998153 ) ) ;
#1518=CARTESIAN_POINT ( 'NONE',  ( -0.8323763977770610722, 4.658724279160015413, 6.176051716722023244 ) ) ;
#1525=CARTESIAN_POINT ( 'NONE',  ( -2.576046737280769605, 4.860232935257343456, 14.43605171672202125 ) ) ;
#1535=CARTESIAN_POINT ( 'NONE',  ( 2.708615832122949652, 5.110351332421781301, 7.263948283277976259 ) ) ;
#1551=CARTESIAN_POINT ( 'NONE',  ( -2.148092372876330813, -4.215868657802593233, 9.659999999999994813 ) ) ;
#1556=CARTESIAN_POINT ( 'NONE',  ( 4.860232935257354114, -2.576046737280751842, 5.163948283277975726 ) ) ;
#1559=CARTESIAN_POINT ( 'NONE',  ( -4.089228379062038066, 4.089228379062022078, 2.099999999999999645 ) ) ;
#1568=CARTESIAN_POINT ( 'NONE',  ( -4.009529358847660596, 2.042957248827953265, 7.559999999999998721 ) ) ;
#1582=CARTESIAN_POINT ( 'NONE',  ( -3.411736077305382420, 3.279728542977939476, 3.096051716722023617 ) ) ;
#1589=CARTESIAN_POINT ( 'NONE',  ( 2.625446233515515537, 5.152728359536502545, 8.259999999999999787 ) ) ;
#1591=CARTESIAN_POINT ( 'NONE',  ( -5.711843387010018702, 0.9046671180729746187, 4.620000000000000107 ) ) ;
#1603=CARTESIAN_POINT ( 'NONE',  ( 0.7039550926810297371, 4.444597532678122853, 8.119999999999999218 ) ) ;
#1606=CARTESIAN_POINT ( 'NONE',  ( -4.900535883036028828, 2.496947748567499126, 7.559999999999998721 ) ) ;
#1609=CARTESIAN_POINT ( 'NONE',  ( -0.9046671180729962680, 5.711843387010016926, 2.379999999999999893 ) ) ;
#1618=CARTESIAN_POINT ( 'NONE',  ( 4.215868657802586128, 2.148092372876346801, 8.539999999999999147 ) ) ;
#1625=( NAMED_UNIT ( * ) PLANE_ANGLE_UNIT ( ) SI_UNIT ( $, .RADIAN. ) );
#1631=CARTESIAN_POINT ( 'NONE',  ( -5.726445515403654873, 0.8124729078101847746, 14.01605171672202310 ) ) ;
#1640=CARTESIAN_POINT ( 'NONE',  ( 4.089228379062037178, -4.089228379062022967, 6.299999999999999822 ) ) ;
#1642=CARTESIAN_POINT ( 'NONE',  ( 4.860232935257354114, -2.576046737280751842, 10.76394828327797626 ) ) ;
#1652=CARTESIAN_POINT ( 'NONE',  ( 4.258245684917310037, 2.064922774268912686, 4.743948283277974909 ) ) ;
#1655=CARTESIAN_POINT ( 'NONE',  ( 0.8603895577212593571, 5.432285873273261068, 8.119999999999999218 ) ) ;
#1666=CARTESIAN_POINT ( 'NONE',  ( 0.6479879772514793856, -4.687928535947285091, 5.583948283277975655 ) ) ;
#1667=UNCERTAINTY_MEASURE_WITH_UNIT (LENGTH_MEASURE( 1.000000000000000082E-05 ), #10273, 'distance_accuracy_value', 'NONE');
#1675=CARTESIAN_POINT ( 'NONE',  ( -0.7401821875142703400, 4.673326407553649808, 5.179999999999999716 ) ) ;
#1680=CARTESIAN_POINT ( 'NONE',  ( 2.122056237541221524, -3.969226411068978777, 7.436051716722023031 ) ) ;
#1690=CARTESIAN_POINT ( 'NONE',  ( 5.152728359536493663, 2.625446233515533745, 0.1399999999999999856 ) ) ;
#1692=CARTESIAN_POINT ( 'NONE',  ( -2.625446233515515981, -5.152728359536500768, 4.059999999999999609 ) ) ;
#1704=CARTESIAN_POINT ( 'NONE',  ( -0.7916369971161423269, -4.430710083317576320, 2.923948283277976401 ) ) ;
#1710=CARTESIAN_POINT ( 'NONE',  ( -5.432285873273256627, -0.8603895577212797852, 1.679999999999999938 ) ) ;
#1714=CARTESIAN_POINT ( 'NONE',  ( 5.432285873273257515, 0.8603895577212793411, 5.879999999999999893 ) ) ;
#1721=CARTESIAN_POINT ( 'NONE',  ( -3.119207202478379681, -3.244753828200550139, 5.196051716722022817 ) ) ;
#1724=CARTESIAN_POINT ( 'NONE',  ( 3.279728542977952799, -3.411736077305369541, 8.103948283277974340 ) ) ;
#1731=CARTESIAN_POINT ( 'NONE',  ( -0.7401821875142703400, 4.673326407553649808, 2.379999999999999893 ) ) ;
#1734=CARTESIAN_POINT ( 'NONE',  ( -3.119207202478379681, -3.244753828200550139, 5.196051716722022817 ) ) ;
#1741=CARTESIAN_POINT ( 'NONE',  ( 0.8603895577212593571, 5.432285873273261068, 5.319999999999999396 ) ) ;
#1742=CARTESIAN_POINT ( 'NONE',  ( 0.9046671180729951578, -5.711843387010016926, 0.9799999999999997602 ) ) ;
#1743=CARTESIAN_POINT ( 'NONE',  ( 5.432285873273257515, 0.8603895577212793411, 0.2799999999999999156 ) ) ;
#1756=CARTESIAN_POINT ( 'NONE',  ( 1.963858260114715870, -4.049832306626327316, -0.1560517167220233370 ) ) ;
#1759=CARTESIAN_POINT ( 'NONE',  ( -2.625446233515515981, -5.152728359536500768, 4.059999999999999609 ) ) ;
#1763=CARTESIAN_POINT ( 'NONE',  ( 2.625446233515515093, 5.152728359536503433, 8.259999999999999787 ) ) ;
#1769=CARTESIAN_POINT ( 'NONE',  ( 3.119207202478379681, 3.244753828200549695, 3.796051716722023350 ) ) ;
#1771=CARTESIAN_POINT ( 'NONE',  ( -3.969226411068985882, 2.122056237541205537, 9.363948283277975904 ) ) ;
#1775=CARTESIAN_POINT ( 'NONE',  ( 5.418398423912711870, 0.9480714621563913758, 6.876051716722023421 ) ) ;
#1786=CARTESIAN_POINT ( 'NONE',  ( -4.089228379062038066, 4.089228379062021190, 2.099999999999999201 ) ) ;
#1787=CARTESIAN_POINT ( 'NONE',  ( -4.173491630687863108, -2.231261971483782691, 5.336051716722022498 ) ) ;
#1795=CARTESIAN_POINT ( 'NONE',  ( -5.432285873273256627, -0.8603895577212797852, 4.479999999999999538 ) ) ;
#1796=CARTESIAN_POINT ( 'NONE',  ( 2.496947748567516889, -4.900535883036019946, 0.8399999999999999689 ) ) ;
#1797=CARTESIAN_POINT ( 'NONE',  ( -5.152728359536494551, -2.625446233515535077, 4.339999999999999858 ) ) ;
#1810=CARTESIAN_POINT ( 'NONE',  ( -3.279728542977953687, 3.411736077305369541, 1.103948283277976561 ) ) ;
#1813=CARTESIAN_POINT ( 'NONE',  ( -2.625446233515515981, -5.152728359536500768, 1.259999999999999787 ) ) ;
#1816=CARTESIAN_POINT ( 'NONE',  ( 4.089228379062037178, -4.089228379062022967, 3.499999999999999112 ) ) ;
#1821=CARTESIAN_POINT ( 'NONE',  ( 4.687928535947288644, -0.6479879772514620662, 1.416051716722023235 ) ) ;
#1823=CARTESIAN_POINT ( 'NONE',  ( -3.279728542977953687, 3.411736077305369541, 3.903948283277975939 ) ) ;
#1827=CARTESIAN_POINT ( 'NONE',  ( -3.826313983664925811, -3.951860609387098489, 5.196051716722022817 ) ) ;
#1834=CARTESIAN_POINT ( 'NONE',  ( -4.687928535947287756, 0.6479879772514611780, 11.21605171672202417 ) ) ;
#1845=CARTESIAN_POINT ( 'NONE',  ( 2.496947748567516889, -4.900535883036019946, 12.03999999999999915 ) ) ;
#1846=CARTESIAN_POINT ( 'NONE',  ( -2.496947748567517333, 4.900535883036019058, 7.839999999999999858 ) ) ;
#1847=CARTESIAN_POINT ( 'NONE',  ( -5.711843387010018702, 0.9046671180729746187, 7.419999999999998153 ) ) ;
#1861=CARTESIAN_POINT ( 'NONE',  ( 1.963858260114715870, -4.049832306626327316, 2.643948283277976596 ) ) ;
#1865=CARTESIAN_POINT ( 'NONE',  ( 0.8603895577212593571, 5.432285873273261068, 10.91999999999999993 ) ) ;
#1867=CARTESIAN_POINT ( 'NONE',  ( -5.711843387010019590, 0.9046671180729746187, 4.620000000000000107 ) ) ;
#1873=CARTESIAN_POINT ( 'NONE',  ( 2.122056237541221524, -3.969226411068978777, 4.636051716722022320 ) ) ;
#1876=CARTESIAN_POINT ( 'NONE',  ( -3.279728542977953687, 3.411736077305369541, 1.103948283277976561 ) ) ;
#1880=CARTESIAN_POINT ( 'NONE',  ( 5.110351332421769754, 2.708615832122969191, 6.736051716722023741 ) ) ;
#1889=CARTESIAN_POINT ( 'NONE',  ( -0.8323763977770610722, 4.658724279160015413, 8.976051716722020402 ) ) ;
#1900=CARTESIAN_POINT ( 'NONE',  ( 5.726445515403654873, -0.8124729078101852187, 4.216051716722023279 ) ) ;
#1902=CARTESIAN_POINT ( 'NONE',  ( 5.152728359536493663, 2.625446233515533745, 5.739999999999997549 ) ) ;
#1903=CARTESIAN_POINT ( 'NONE',  ( -5.432285873273256627, -0.8603895577212797852, 7.279999999999999361 ) ) ;
#1915=CARTESIAN_POINT ( 'NONE',  ( -4.658724279160018078, 0.8323763977770419764, 6.423948283277978177 ) ) ;
#1918=CARTESIAN_POINT ( 'NONE',  ( 5.432285873273257515, 0.8603895577212793411, 11.47999999999999865 ) ) ;
#1920=CARTESIAN_POINT ( 'NONE',  ( 2.625446233515515093, 5.152728359536503433, 5.459999999999999076 ) ) ;
#1925=CARTESIAN_POINT ( 'NONE',  ( 4.687928535947288644, -0.6479879772514620662, 12.61605171672202097 ) ) ;
#1928=CARTESIAN_POINT ( 'NONE',  ( 4.023224611898322145, -4.155232146225737111, -0.2960517167220233503 ) ) ;
#1932=CARTESIAN_POINT ( 'NONE',  ( 2.542276634908080535, 5.195105386651229118, 6.456051716722022604 ) ) ;
#1937=CARTESIAN_POINT ( 'NONE',  ( 2.042957248827968808, -4.009529358847652603, 12.03999999999999915 ) ) ;
#1939=CARTESIAN_POINT ( 'NONE',  ( -2.148092372876330813, -4.215868657802593233, 1.259999999999999787 ) ) ;
#1949=CARTESIAN_POINT ( 'NONE',  ( 0.9046671180729951578, -5.711843387010016926, 12.17999999999999439 ) ) ;
#1950=CARTESIAN_POINT ( 'NONE',  ( -3.889087296526005044, -3.889087296526019255, 1.399999999999999689 ) ) ;
#1952=CARTESIAN_POINT ( 'NONE',  ( 4.089228379062037178, -4.089228379062022967, 9.099999999999999645 ) ) ;
#1966=CARTESIAN_POINT ( 'NONE',  ( 5.195105386651219348, 2.542276634908100075, -0.8560517167220232926 ) ) ;
#1979=CARTESIAN_POINT ( 'NONE',  ( 3.411736077305382420, -3.279728542977940364, 10.09605171672202140 ) ) ;
#1981=CARTESIAN_POINT ( 'NONE',  ( -0.6479879772514802738, 4.687928535947285091, 9.783948283277975833 ) ) ;
#1985=CARTESIAN_POINT ( 'NONE',  ( 0.7727076532861471003, 5.446173322633805824, 9.116051716722020970 ) ) ;
#1989=CARTESIAN_POINT ( 'NONE',  ( -3.345732310141667831, 3.345732310141653620, 7.699999999999998401 ) ) ;
#1992=CARTESIAN_POINT ( 'NONE',  ( 3.119207202478379681, 3.244753828200549695, 14.99605171672202175 ) ) ;
#2002=CARTESIAN_POINT ( 'NONE',  ( -0.9046671180729963790, 5.711843387010016926, 10.77999999999999936 ) ) ;
#2003=CARTESIAN_POINT ( 'NONE',  ( 5.432285873273257515, 0.8603895577212793411, 8.679999999999997939 ) ) ;
#2004=CARTESIAN_POINT ( 'NONE',  ( 2.496947748567516889, -4.900535883036019946, 6.439999999999999503 ) ) ;
#2015=CARTESIAN_POINT ( 'NONE',  ( 1.963858260114715870, -4.049832306626327316, 8.243948283277976685 ) ) ;
#2019=CARTESIAN_POINT ( 'NONE',  ( -4.900535883036028828, 2.496947748567499126, 13.15999999999999837 ) ) ;
#2021=CARTESIAN_POINT ( 'NONE',  ( -2.625446233515515537, -5.152728359536502545, 12.45999999999999730 ) ) ;
#2026=CARTESIAN_POINT ( 'NONE',  ( -3.411736077305382420, 3.279728542977939476, 8.696051716722022817 ) ) ;
#2031=CARTESIAN_POINT ( 'NONE',  ( -2.231261971483764484, -4.173491630687871101, 11.46394828327797555 ) ) ;
#2041=CARTESIAN_POINT ( 'NONE',  ( -4.673326407553653361, 0.7401821875142517992, 7.419999999999999041 ) ) ;
#2044=CARTESIAN_POINT ( 'NONE',  ( 0.7401821875142697849, -4.673326407553650697, 0.9799999999999997602 ) ) ;
#2055=CARTESIAN_POINT ( 'NONE',  ( -0.7727076532861475444, -5.446173322633804048, 4.916051716722023457 ) ) ;
#2056=CARTESIAN_POINT ( 'NONE',  ( -5.152728359536494551, -2.625446233515535077, 9.939999999999994174 ) ) ;
#2058=CARTESIAN_POINT ( 'NONE',  ( -5.432285873273256627, -0.8603895577212797852, 10.07999999999999829 ) ) ;
#2070=CARTESIAN_POINT ( 'NONE',  ( -3.969226411068985882, 2.122056237541205537, 6.563948283277975193 ) ) ;
#2073=CARTESIAN_POINT ( 'NONE',  ( -5.152728359536494551, -2.625446233515535077, 12.73999999999999488 ) ) ;
#2075=CARTESIAN_POINT ( 'NONE',  ( 0.9046671180729953798, -5.711843387010016926, 12.17999999999999616 ) ) ;
#2080=CARTESIAN_POINT ( 'NONE',  ( 3.345732310141667387, -3.345732310141653620, 0.6999999999999997335 ) ) ;
#2082=CARTESIAN_POINT ( 'NONE',  ( -0.8124729078102072011, 5.726445515403652209, 4.183948283277976188 ) ) ;
#2093=CARTESIAN_POINT ( 'NONE',  ( -2.042957248827969252, 4.009529358847651714, 7.839999999999999858 ) ) ;
#2096=CARTESIAN_POINT ( 'NONE',  ( -3.181980515339458027, -3.181980515339470905, 4.200000000000000178 ) ) ;
#2101=AXIS2_PLACEMENT_3D ( 'NONE', #7090, #5610, #4547 ) ;
#2105=CARTESIAN_POINT ( 'NONE',  ( -5.110351332421769754, -2.708615832122969191, 5.336051716722022498 ) ) ;
#2111=( NAMED_UNIT ( * ) PLANE_ANGLE_UNIT ( ) SI_UNIT ( $, .RADIAN. ) );
#2119=CARTESIAN_POINT ( 'NONE',  ( -0.6479879772514802738, 4.687928535947285091, 6.983948283277976010 ) ) ;
#2120=ORIENTED_EDGE ( 'NONE', *, *, #9280, .F. ) ;
#2133=CARTESIAN_POINT ( 'NONE',  ( 4.430710083317573655, 0.7916369971161595354, 9.676051716722021467 ) ) ;
#2137=CARTESIAN_POINT ( 'NONE',  ( 4.258245684917310037, 2.064922774268912686, 10.34394828327797633 ) ) ;
#2148=CARTESIAN_POINT ( 'NONE',  ( -2.148092372876330813, -4.215868657802593233, 4.059999999999999609 ) ) ;
#2156=CARTESIAN_POINT ( 'NONE',  ( -2.576046737280769605, 4.860232935257343456, 6.036051716722022675 ) ) ;
#2169=CARTESIAN_POINT ( 'NONE',  ( 4.023224611898322145, -4.155232146225737111, 8.103948283277974340 ) ) ;
#2176=CARTESIAN_POINT ( 'NONE',  ( -4.089228379062038066, 4.089228379062022078, 13.29999999999999716 ) ) ;
#2181=CARTESIAN_POINT ( 'NONE',  ( -0.7039550926810301812, -4.444597532678121965, 3.919999999999999929 ) ) ;
#2184=CARTESIAN_POINT ( 'NONE',  ( 4.860232935257354114, -2.576046737280751842, 10.76394828327797626 ) ) ;
#2194=VERTEX_POINT ( 'NONE', #7758 ) ;
#2199=CARTESIAN_POINT ( 'NONE',  ( -3.244753828200538148, -3.119207202478392116, 0.4039482832779765498 ) ) ;
#2208=CARTESIAN_POINT ( 'NONE',  ( -2.542276634908081423, -5.195105386651227342, 5.056051716722023137 ) ) ;
#2214=SURFACE_SIDE_STYLE ('',( #674 ) ) ;
#2226=CARTESIAN_POINT ( 'NONE',  ( 2.417848759854264618, -4.940838830814695548, 8.243948283277976685 ) ) ;
#2238=CARTESIAN_POINT ( 'NONE',  ( 0.7039550926810297371, 4.444597532678122853, 2.519999999999999574 ) ) ;
#2240=CARTESIAN_POINT ( 'NONE',  ( -4.860232935257354114, 2.576046737280751842, 6.563948283277975193 ) ) ;
#2251=CARTESIAN_POINT ( 'NONE',  ( 4.444597532678119300, 0.7039550926810472786, 11.47999999999999865 ) ) ;
#2260=CARTESIAN_POINT ( 'NONE',  ( -5.726445515403654873, 0.8124729078101847746, 8.416051716722021681 ) ) ;
#2261=CARTESIAN_POINT ( 'NONE',  ( 2.625446233515515537, 5.152728359536502545, 13.85999999999999766 ) ) ;
#2264=CARTESIAN_POINT ( 'NONE',  ( 3.826313983664925811, 3.951860609387098044, 14.99605171672202175 ) ) ;
#2274=CARTESIAN_POINT ( 'NONE',  ( 4.860232935257354114, -2.576046737280751842, 5.163948283277975726 ) ) ;
#2288=CARTESIAN_POINT ( 'NONE',  ( -4.444597532678119300, -0.7039550926810477227, 10.07999999999999829 ) ) ;
#2292=CARTESIAN_POINT ( 'NONE',  ( 3.951860609387084722, 3.826313983664940022, 13.00394828327797470 ) ) ;
#2306=CARTESIAN_POINT ( 'NONE',  ( 2.148092372876330369, 4.215868657802593233, 11.05999999999999872 ) ) ;
#2313=CARTESIAN_POINT ( 'NONE',  ( -4.049832306626335310, 1.963858260114700327, 8.556051716722022249 ) ) ;
#2318=CARTESIAN_POINT ( 'NONE',  ( 0.9968613283357860011, -5.697241258616382531, 13.17605171672201969 ) ) ;
#2328=CARTESIAN_POINT ( 'NONE',  ( 5.195105386651219348, 2.542276634908100075, 1.943948283277976419 ) ) ;
#2340=CARTESIAN_POINT ( 'NONE',  ( -4.444597532678119300, -0.7039550926810477227, 4.479999999999999538 ) ) ;
#2342=CARTESIAN_POINT ( 'NONE',  ( 0.8124729078102063129, -5.726445515403652209, 5.583948283277975655 ) ) ;
#2346=CARTESIAN_POINT ( 'NONE',  ( -5.711843387010019590, 0.9046671180729746187, 1.819999999999999618 ) ) ;
#2356=CARTESIAN_POINT ( 'NONE',  ( -0.7401821875142701179, 4.673326407553649808, 7.979999999999999538 ) ) ;
#2357=APPLICATION_CONTEXT ( 'automotive_design' ) ;
#2360=EDGE_LOOP ( 'NONE', ( #4693, #6871 ) ) ;
#2370=CARTESIAN_POINT ( 'NONE',  ( -5.110351332421769754, -2.708615832122969191, 10.93605171672202125 ) ) ;
#2378=CARTESIAN_POINT ( 'NONE',  ( -0.8603895577212598011, -5.432285873273260179, 6.719999999999999751 ) ) ;
#2380=CARTESIAN_POINT ( 'NONE',  ( -4.900535883036028828, 2.496947748567499126, 1.959999999999999964 ) ) ;
#2397=CARTESIAN_POINT ( 'NONE',  ( -0.7401821875142701179, 4.673326407553649808, 5.179999999999999716 ) ) ;
#2401=CARTESIAN_POINT ( 'NONE',  ( 2.708615832122949652, 5.110351332421781301, 10.06394828327797519 ) ) ;
#2406=CARTESIAN_POINT ( 'NONE',  ( 2.496947748567516889, -4.900535883036019946, 0.8399999999999999689 ) ) ;
#2414=CARTESIAN_POINT ( 'NONE',  ( 4.658724279160018966, -0.8323763977770426425, -0.5760517167220230439 ) ) ;
#2424=CARTESIAN_POINT ( 'NONE',  ( -2.148092372876330813, -4.215868657802594122, 1.259999999999999787 ) ) ;
#2427=CARTESIAN_POINT ( 'NONE',  ( -4.173491630687863108, -2.231261971483782691, 2.536051716722023119 ) ) ;
#2435=CARTESIAN_POINT ( 'NONE',  ( 5.711843387010018702, -0.9046671180729751738, 0.4199999999999999289 ) ) ;
#2437=CARTESIAN_POINT ( 'NONE',  ( 0.8124729078102063129, -5.726445515403652209, 11.18394828327797441 ) ) ;
#2451=CARTESIAN_POINT ( 'NONE',  ( -4.658724279160018078, 0.8323763977770419764, 3.623948283277976135 ) ) ;
#2454=CARTESIAN_POINT ( 'NONE',  ( -2.496947748567517333, 4.900535883036019058, 7.839999999999999858 ) ) ;
#2458=CARTESIAN_POINT ( 'NONE',  ( 5.152728359536493663, 2.625446233515533745, 2.939999999999999503 ) ) ;
#2468=CARTESIAN_POINT ( 'NONE',  ( 3.244753828200538148, 3.119207202478391672, 4.603948283277976117 ) ) ;
#2476=CARTESIAN_POINT ( 'NONE',  ( -4.673326407553653361, 0.7401821875142517992, 4.620000000000000107 ) ) ;
#2480=CARTESIAN_POINT ( 'NONE',  ( 3.119207202478379681, 3.244753828200549695, 9.396051716722022107 ) ) ;
#2487=CARTESIAN_POINT ( 'NONE',  ( 3.889087296526005488, 3.889087296526018811, 2.799999999999999378 ) ) ;
#2490=CARTESIAN_POINT ( 'NONE',  ( 4.900535883036028828, -2.496947748567499126, 3.359999999999999876 ) ) ;
#2501=CARTESIAN_POINT ( 'NONE',  ( 0.7916369971161419938, 4.430710083317576320, 1.523948283277976268 ) ) ;
#2504=CARTESIAN_POINT ( 'NONE',  ( 5.711843387010018702, -0.9046671180729751738, 0.4199999999999999289 ) ) ;
#2512=CARTESIAN_POINT ( 'NONE',  ( 0.8323763977770604061, -4.658724279160015413, 4.776051716722021112 ) ) ;
#2515=CARTESIAN_POINT ( 'NONE',  ( 4.658724279160018966, -0.8323763977770426425, 7.823948283277974980 ) ) ;
#2522=CARTESIAN_POINT ( 'NONE',  ( -2.148092372876330813, -4.215868657802594122, 4.059999999999999609 ) ) ;
#2526=CARTESIAN_POINT ( 'NONE',  ( -4.049832306626335310, 1.963858260114700327, 11.35605171672202296 ) ) ;
#2536=CARTESIAN_POINT ( 'NONE',  ( -4.089228379062038066, 4.089228379062021190, 4.900000000000000355 ) ) ;
#2537=CARTESIAN_POINT ( 'NONE',  ( -0.8603895577212598011, -5.432285873273260179, 6.719999999999999751 ) ) ;
#2538=CARTESIAN_POINT ( 'NONE',  ( -2.417848759854264618, 4.940838830814694660, 9.643948283277975264 ) ) ;
#2552=CARTESIAN_POINT ( 'NONE',  ( 0.6479879772514793856, -4.687928535947285091, -0.01605171672202330979 ) ) ;
#2556=CARTESIAN_POINT ( 'NONE',  ( 0.8603895577212593571, 5.432285873273261068, 2.519999999999999574 ) ) ;
#2561=CARTESIAN_POINT ( 'NONE',  ( -0.8603895577212598011, -5.432285873273260179, 6.719999999999999751 ) ) ;
#2567=CARTESIAN_POINT ( 'NONE',  ( -3.411736077305382420, 3.279728542977939476, 5.896051716722023883 ) ) ;
#2569=CARTESIAN_POINT ( 'NONE',  ( 4.458484982038663169, 0.6162731882459350219, 7.683948283277975300 ) ) ;
#2572=CARTESIAN_POINT ( 'NONE',  ( -5.110351332421769754, -2.708615832122969191, 5.336051716722022498 ) ) ;
#2577=CARTESIAN_POINT ( 'NONE',  ( -4.444597532678119300, -0.7039550926810477227, 4.479999999999999538 ) ) ;
#2580=CARTESIAN_POINT ( 'NONE',  ( -3.119207202478379681, -3.244753828200550139, 10.79605171672202246 ) ) ;
#2590=CARTESIAN_POINT ( 'NONE',  ( -5.711843387010018702, 0.9046671180729746187, 1.819999999999999396 ) ) ;
#2592=CARTESIAN_POINT ( 'NONE',  ( 5.432285873273257515, 0.8603895577212793411, 0.2799999999999999156 ) ) ;
#2593=CARTESIAN_POINT ( 'NONE',  ( -0.8124729078102072011, 5.726445515403652209, 9.783948283277975833 ) ) ;
#2606=CARTESIAN_POINT ( 'NONE',  ( -3.244753828200538148, -3.119207202478392116, 0.4039482832779765498 ) ) ;
#2611=CARTESIAN_POINT ( 'NONE',  ( -4.089228379062038066, 4.089228379062021190, 2.099999999999999201 ) ) ;
#2613=CARTESIAN_POINT ( 'NONE',  ( -3.889087296526005044, -3.889087296526019255, 6.999999999999999112 ) ) ;
#2617=CARTESIAN_POINT ( 'NONE',  ( 3.411736077305382420, -3.279728542977940364, 1.696051716722023484 ) ) ;
#2621=CARTESIAN_POINT ( 'NONE',  ( 1.963858260114715870, -4.049832306626327316, 2.643948283277976596 ) ) ;
#2624=CARTESIAN_POINT ( 'NONE',  ( -0.9968613283357868893, 5.697241258616382531, 3.376051716722022977 ) ) ;
#2631=CARTESIAN_POINT ( 'NONE',  ( 4.173491630687861331, 2.231261971483781359, 12.33605171672202339 ) ) ;
#2640=CARTESIAN_POINT ( 'NONE',  ( 5.711843387010018702, -0.9046671180729751738, 11.61999999999999922 ) ) ;
#2642=CARTESIAN_POINT ( 'NONE',  ( -5.711843387010018702, 0.9046671180729746187, 7.419999999999998153 ) ) ;
#2643=CARTESIAN_POINT ( 'NONE',  ( -2.496947748567517333, 4.900535883036019058, 7.839999999999999858 ) ) ;
#2656=CARTESIAN_POINT ( 'NONE',  ( -2.231261971483764484, -4.173491630687871101, 0.2639482832779765920 ) ) ;
#2659=CARTESIAN_POINT ( 'NONE',  ( -3.889087296526005044, -3.889087296526019255, 12.59999999999999787 ) ) ;
#2661=CARTESIAN_POINT ( 'NONE',  ( 5.711843387010019590, -0.9046671180729753958, 11.61999999999999922 ) ) ;
#2666=CARTESIAN_POINT ( 'NONE',  ( 2.122056237541221524, -3.969226411068978777, 1.836051716722023386 ) ) ;
#2668=CARTESIAN_POINT ( 'NONE',  ( -4.658724279160018078, 0.8323763977770419764, 3.623948283277976135 ) ) ;
#2672=CARTESIAN_POINT ( 'NONE',  ( -2.542276634908081423, -5.195105386651227342, 2.256051716722022871 ) ) ;
#2677=CARTESIAN_POINT ( 'NONE',  ( 0.7401821875142697849, -4.673326407553650697, 12.17999999999999616 ) ) ;
#2679=CARTESIAN_POINT ( 'NONE',  ( -2.064922774268895811, -4.258245684917318918, 5.056051716722023137 ) ) ;
#2688=CARTESIAN_POINT ( 'NONE',  ( 5.110351332421769754, 2.708615832122969191, 1.136051716722023208 ) ) ;
#2689=CARTESIAN_POINT ( 'NONE',  ( -2.496947748567517333, 4.900535883036019058, 2.239999999999999769 ) ) ;
#2690=CARTESIAN_POINT ( 'NONE',  ( -5.432285873273256627, -0.8603895577212797852, 12.87999999999999901 ) ) ;
#2702=CARTESIAN_POINT ( 'NONE',  ( -0.6479879772514802738, 4.687928535947285091, 12.58394828327797477 ) ) ;
#2707=CARTESIAN_POINT ( 'NONE',  ( 0.9046671180729951578, -5.711843387010016926, 9.379999999999995453 ) ) ;
#2710=CARTESIAN_POINT ( 'NONE',  ( 4.089228379062037178, -4.089228379062022967, 11.89999999999999858 ) ) ;
#2716=CARTESIAN_POINT ( 'NONE',  ( -0.7039550926810301812, -4.444597532678121965, 1.119999999999999885 ) ) ;
#2719=CARTESIAN_POINT ( 'NONE',  ( -1.963858260114716980, 4.049832306626327316, 12.44394828327797597 ) ) ;
#2724=CARTESIAN_POINT ( 'NONE',  ( -5.418398423912711870, -0.9480714621563917088, 8.276051716722021112 ) ) ;
#2730=CARTESIAN_POINT ( 'NONE',  ( 4.009529358847659708, -2.042957248827953709, 11.75999999999999979 ) ) ;
#2735=CARTESIAN_POINT ( 'NONE',  ( 2.148092372876330369, 4.215868657802593233, 2.659999999999998366 ) ) ;
#2744=CARTESIAN_POINT ( 'NONE',  ( 0.9968613283357860011, -5.697241258616382531, 4.776051716722021112 ) ) ;
#2745=CARTESIAN_POINT ( 'NONE',  ( 5.152728359536493663, 2.625446233515533745, 2.939999999999999059 ) ) ;
#2746=CARTESIAN_POINT ( 'NONE',  ( -2.625446233515515981, -5.152728359536500768, 6.859999999999999432 ) ) ;
#2757=CARTESIAN_POINT ( 'NONE',  ( 3.951860609387084722, 3.826313983664940022, -0.9960517167220231949 ) ) ;
#2761=CARTESIAN_POINT ( 'NONE',  ( -5.432285873273256627, -0.8603895577212797852, 10.07999999999999829 ) ) ;
#2763=CARTESIAN_POINT ( 'NONE',  ( 2.496947748567516889, -4.900535883036019946, 6.439999999999999503 ) ) ;
#2769=CARTESIAN_POINT ( 'NONE',  ( -3.181980515339458027, -3.181980515339470905, 1.399999999999999689 ) ) ;
#2771=CARTESIAN_POINT ( 'NONE',  ( 4.658724279160018966, -0.8323763977770426425, 10.62394828327797569 ) ) ;
#2775=CARTESIAN_POINT ( 'NONE',  ( -4.155232146225753098, 4.023224611898306158, 3.096051716722023617 ) ) ;
#2781=CARTESIAN_POINT ( 'NONE',  ( 0.7401821875142697849, -4.673326407553650697, 9.379999999999997229 ) ) ;
#2783=CARTESIAN_POINT ( 'NONE',  ( 2.148092372876330369, 4.215868657802593233, 5.459999999999997300 ) ) ;
#2791=CARTESIAN_POINT ( 'NONE',  ( 3.826313983664925811, 3.951860609387098044, 0.9960517167220231949 ) ) ;
#2793=CARTESIAN_POINT ( 'NONE',  ( -2.496947748567517333, 4.900535883036019058, 10.63999999999999879 ) ) ;
#2795=CARTESIAN_POINT ( 'NONE',  ( 0.9046671180729951578, -5.711843387010016926, 12.17999999999999439 ) ) ;
#2810=CARTESIAN_POINT ( 'NONE',  ( 2.417848759854264618, -4.940838830814695548, -0.1560517167220233370 ) ) ;
#2814=CARTESIAN_POINT ( 'NONE',  ( 3.889087296526005488, 3.889087296526018811, 11.19999999999999751 ) ) ;
#2822=CARTESIAN_POINT ( 'NONE',  ( 4.049832306626335310, -1.963858260114701215, 12.75605171672202331 ) ) ;
#2824=CARTESIAN_POINT ( 'NONE',  ( 3.951860609387084722, 3.826313983664940022, 1.803948283277976516 ) ) ;
#2832=CARTESIAN_POINT ( 'NONE',  ( 4.215868657802586128, 2.148092372876346801, 8.539999999999999147 ) ) ;
#2833=CARTESIAN_POINT ( 'NONE',  ( -4.444597532678119300, -0.7039550926810477227, 4.479999999999999538 ) ) ;
#2842=CARTESIAN_POINT ( 'NONE',  ( -4.900535883036028828, 2.496947748567499126, 13.15999999999999837 ) ) ;
#2843=CARTESIAN_POINT ( 'NONE',  ( -4.089228379062038066, 4.089228379062021190, 13.29999999999999538 ) ) ;
#2844=CARTESIAN_POINT ( 'NONE',  ( -2.625446233515515981, -5.152728359536500768, 9.659999999999994813 ) ) ;
#2856=CARTESIAN_POINT ( 'NONE',  ( -1.963858260114716980, 4.049832306626327316, 12.44394828327797597 ) ) ;
#2861=CARTESIAN_POINT ( 'NONE',  ( 3.889087296526005488, 3.889087296526018811, 13.99999999999999822 ) ) ;
#2868=CARTESIAN_POINT ( 'NONE',  ( -3.119207202478379681, -3.244753828200550139, 13.59605171672202140 ) ) ;
#2872=CARTESIAN_POINT ( 'NONE',  ( -4.023224611898323033, 4.155232146225737111, 3.903948283277975939 ) ) ;
#2882=CARTESIAN_POINT ( 'NONE',  ( -0.7401821875142703400, 4.673326407553649808, 13.57999999999999652 ) ) ;
#2885=CARTESIAN_POINT ( 'NONE',  ( -3.345732310141667831, 3.345732310141653620, 2.099999999999999201 ) ) ;
#2897=CARTESIAN_POINT ( 'NONE',  ( -5.726445515403654873, 0.8124729078101847746, 11.21605171672202417 ) ) ;
#2898=CARTESIAN_POINT ( 'NONE',  ( 5.152728359536493663, 2.625446233515533745, 8.539999999999999147 ) ) ;
#2915=CARTESIAN_POINT ( 'NONE',  ( -3.279728542977953687, 3.411736077305369541, 6.703948283277976650 ) ) ;
#2921=CARTESIAN_POINT ( 'NONE',  ( -5.432285873273256627, -0.8603895577212797852, 12.87999999999999901 ) ) ;
#2927=CARTESIAN_POINT ( 'NONE',  ( 0.7401821875142697849, -4.673326407553650697, 0.9799999999999997602 ) ) ;
#2929=CARTESIAN_POINT ( 'NONE',  ( 2.708615832122949652, 5.110351332421781301, 4.463948283277976437 ) ) ;
#2943=CARTESIAN_POINT ( 'NONE',  ( -2.122056237541221968, 3.969226411068977889, 14.43605171672202125 ) ) ;
#2952=CARTESIAN_POINT ( 'NONE',  ( -0.9968613283357868893, 5.697241258616382531, 8.976051716722020402 ) ) ;
#2966=CARTESIAN_POINT ( 'NONE',  ( -2.417848759854264618, 4.940838830814694660, 1.243948283277976463 ) ) ;
#2973=CARTESIAN_POINT ( 'NONE',  ( -3.889087296526005044, -3.889087296526019255, 12.59999999999999787 ) ) ;
#2980=CARTESIAN_POINT ( 'NONE',  ( 3.181980515339458471, 3.181980515339470461, 8.400000000000000355 ) ) ;
#2983=CARTESIAN_POINT ( 'NONE',  ( -0.8124729078102072011, 5.726445515403652209, 6.983948283277976010 ) ) ;
#2995=CARTESIAN_POINT ( 'NONE',  ( -2.148092372876330813, -4.215868657802593233, 9.659999999999994813 ) ) ;
#3004=CARTESIAN_POINT ( 'NONE',  ( -0.9968613283357868893, 5.697241258616382531, 11.77605171672202289 ) ) ;
#3010=SHAPE_REPRESENTATION_RELATIONSHIP ( 'NONE' , 'NONE' ,  #7608, #6736 ) ;
#3017=CARTESIAN_POINT ( 'NONE',  ( -4.023224611898323033, 4.155232146225737111, 1.103948283277976561 ) ) ;
#3022=CARTESIAN_POINT ( 'NONE',  ( -5.711843387010019590, 0.9046671180729746187, 13.01999999999999602 ) ) ;
#3027=CARTESIAN_POINT ( 'NONE',  ( -2.148092372876330813, -4.215868657802593233, 4.059999999999999609 ) ) ;
#3030=CARTESIAN_POINT ( 'NONE',  ( -0.8124729078102072011, 5.726445515403652209, 9.783948283277975833 ) ) ;
#3046=CARTESIAN_POINT ( 'NONE',  ( 2.042957248827968808, -4.009529358847652603, 9.240000000000000213 ) ) ;
#3052=SURFACE_STYLE_FILL_AREA ( #7877 ) ;
#3055=CARTESIAN_POINT ( 'NONE',  ( -5.418398423912711870, -0.9480714621563917088, 11.07605171672202182 ) ) ;
#3061=CARTESIAN_POINT ( 'NONE',  ( 5.418398423912711870, 0.9480714621563913758, 12.47605171672202218 ) ) ;
#3071=CARTESIAN_POINT ( 'NONE',  ( -3.951860609387083834, -3.826313983664940466, 8.803948283277977183 ) ) ;
#3082=CARTESIAN_POINT ( 'NONE',  ( 3.345732310141667387, -3.345732310141653620, 3.499999999999998668 ) ) ;
#3084=CARTESIAN_POINT ( 'NONE',  ( 0.9480714621563713917, 5.418398423912717199, 9.923948283277976401 ) ) ;
#3096=CARTESIAN_POINT ( 'NONE',  ( -0.7039550926810301812, -4.444597532678121965, 9.519999999999999574 ) ) ;
#3106=CARTESIAN_POINT ( 'NONE',  ( -5.418398423912711870, -0.9480714621563917088, 8.276051716722021112 ) ) ;
#3110=CARTESIAN_POINT ( 'NONE',  ( 2.576046737280769605, -4.860232935257343456, 10.23605171672202374 ) ) ;
#3119=CARTESIAN_POINT ( 'NONE',  ( -5.195105386651219348, -2.542276634908102295, 3.343948283277975886 ) ) ;
#3133=CARTESIAN_POINT ( 'NONE',  ( 4.673326407553653361, -0.7401821875142523544, 8.820000000000000284 ) ) ;
#3135=CARTESIAN_POINT ( 'NONE',  ( -4.860232935257354114, 2.576046737280751842, 12.16394828327797661 ) ) ;
#3151=CARTESIAN_POINT ( 'NONE',  ( 3.244753828200538148, 3.119207202478391672, -0.9960517167220231949 ) ) ;
#3152=PRODUCT_DEFINITION_CONTEXT ( 'detailed design', #2357, 'design' ) ;
#3157=( NAMED_UNIT ( * ) SI_UNIT ( $, .STERADIAN. ) SOLID_ANGLE_UNIT ( ) );
#3163=CARTESIAN_POINT ( 'NONE',  ( 5.110351332421769754, 2.708615832122969191, 9.536051716722020899 ) ) ;
#3170=CARTESIAN_POINT ( 'NONE',  ( -3.889087296526005044, -3.889087296526019255, 6.999999999999999112 ) ) ;
#3172=CARTESIAN_POINT ( 'NONE',  ( -4.023224611898323033, 4.155232146225737111, 3.903948283277975939 ) ) ;
#3185=CARTESIAN_POINT ( 'NONE',  ( -2.148092372876330813, -4.215868657802593233, 6.859999999999999432 ) ) ;
#3190=CARTESIAN_POINT ( 'NONE',  ( 4.860232935257354114, -2.576046737280751842, 7.963948283277976437 ) ) ;
#3202=CARTESIAN_POINT ( 'NONE',  ( 0.7401821875142697849, -4.673326407553650697, 9.379999999999995453 ) ) ;
#3213=CARTESIAN_POINT ( 'NONE',  ( -5.418398423912711870, -0.9480714621563917088, 13.87605171672202253 ) ) ;
#3221=CARTESIAN_POINT ( 'NONE',  ( 0.9046671180729951578, -5.711843387010016926, 0.9799999999999997602 ) ) ;
#3223=CARTESIAN_POINT ( 'NONE',  ( -5.697241258616385196, 0.9968613283357647958, 9.223948283277977112 ) ) ;
#3240=CARTESIAN_POINT ( 'NONE',  ( 4.009529358847659708, -2.042957248827953709, 11.75999999999999979 ) ) ;
#3244=CARTESIAN_POINT ( 'NONE',  ( -4.900535883036028828, 2.496947748567499126, 1.959999999999999964 ) ) ;
#3255=CARTESIAN_POINT ( 'NONE',  ( 2.231261971483764484, 4.173491630687871101, 1.663948283277976392 ) ) ;
#3266=CARTESIAN_POINT ( 'NONE',  ( -3.181980515339458027, -3.181980515339470905, 1.399999999999999689 ) ) ;
#3269=CARTESIAN_POINT ( 'NONE',  ( -5.418398423912711870, -0.9480714621563917088, 11.07605171672202182 ) ) ;
#3278=CARTESIAN_POINT ( 'NONE',  ( 4.089228379062037178, -4.089228379062022967, 0.6999999999999997335 ) ) ;
#3280=CARTESIAN_POINT ( 'NONE',  ( -5.432285873273256627, -0.8603895577212797852, 1.679999999999999938 ) ) ;
#3290=CARTESIAN_POINT ( 'NONE',  ( 4.258245684917310037, 2.064922774268912686, -0.8560517167220232926 ) ) ;
#3293=CARTESIAN_POINT ( 'NONE',  ( 5.152728359536493663, 2.625446233515533745, 8.539999999999999147 ) ) ;
#3296=CARTESIAN_POINT ( 'NONE',  ( 3.181980515339458471, 3.181980515339470461, 3.651811961182260059E-17 ) ) ;
#3300=CARTESIAN_POINT ( 'NONE',  ( -2.625446233515515981, -5.152728359536500768, 1.259999999999999787 ) ) ;
#3303=CARTESIAN_POINT ( 'NONE',  ( 4.049832306626335310, -1.963858260114701215, 1.556051716722023581 ) ) ;
#3308=CARTESIAN_POINT ( 'NONE',  ( 4.658724279160018966, -0.8323763977770426425, 2.223948283277975779 ) ) ;
#3317=CARTESIAN_POINT ( 'NONE',  ( -4.009529358847660596, 2.042957248827953265, 1.959999999999999964 ) ) ;
#3322=CARTESIAN_POINT ( 'NONE',  ( 4.173491630687861331, 2.231261971483781359, 9.536051716722020899 ) ) ;
#3327=DIRECTION ( 'NONE',  ( 0.7043149233066460235, -0.7043149233066438031, 0.08877487040322794287 ) ) ;
#3329=CARTESIAN_POINT ( 'NONE',  ( -4.900535883036028828, 2.496947748567499126, 4.759999999999999787 ) ) ;
#3330=CARTESIAN_POINT ( 'NONE',  ( -5.711843387010018702, 0.9046671180729746187, 1.819999999999999396 ) ) ;
#3331=CARTESIAN_POINT ( 'NONE',  ( 3.889087296526005488, 3.889087296526018811, -3.866961113726609188E-17 ) ) ;
#3341=CARTESIAN_POINT ( 'NONE',  ( 0.7039550926810297371, 4.444597532678122853, 13.71999999999999886 ) ) ;
#3344=CARTESIAN_POINT ( 'NONE',  ( 2.496947748567516889, -4.900535883036019946, 9.240000000000000213 ) ) ;
#3348=CARTESIAN_POINT ( 'NONE',  ( 3.889087296526005488, 3.889087296526018811, 11.19999999999999751 ) ) ;
#3353=CARTESIAN_POINT ( 'NONE',  ( 4.173491630687861331, 2.231261971483781359, 6.736051716722023741 ) ) ;
#3355=CARTESIAN_POINT ( 'NONE',  ( -4.458484982038663169, -0.6162731882459353550, 6.283948283277974944 ) ) ;
#3359=CARTESIAN_POINT ( 'NONE',  ( 2.576046737280769605, -4.860232935257343456, 7.436051716722023031 ) ) ;
#3365=CARTESIAN_POINT ( 'NONE',  ( 0.7039550926810297371, 4.444597532678122853, 5.319999999999999396 ) ) ;
#3369=CARTESIAN_POINT ( 'NONE',  ( -2.064922774268895811, -4.258245684917318918, 7.856051716722022071 ) ) ;
#3380=CARTESIAN_POINT ( 'NONE',  ( 5.711843387010018702, -0.9046671180729751738, 6.019999999999999574 ) ) ;
#3381=CARTESIAN_POINT ( 'NONE',  ( 5.432285873273257515, 0.8603895577212793411, 5.879999999999999893 ) ) ;
#3382=CARTESIAN_POINT ( 'NONE',  ( -5.446173322633801384, -0.7727076532861678615, 9.083948283277974767 ) ) ;
#3396=CARTESIAN_POINT ( 'NONE',  ( 4.673326407553653361, -0.7401821875142523544, 11.61999999999999922 ) ) ;
#3401=CARTESIAN_POINT ( 'NONE',  ( -5.432285873273256627, -0.8603895577212797852, 7.279999999999999361 ) ) ;
#3406=CARTESIAN_POINT ( 'NONE',  ( 5.152728359536493663, 2.625446233515533745, 5.739999999999998437 ) ) ;
#3412=CARTESIAN_POINT ( 'NONE',  ( -4.049832306626335310, 1.963858260114700327, 5.756051716722022427 ) ) ;
#3414=CARTESIAN_POINT ( 'NONE',  ( -0.6479879772514802738, 4.687928535947285091, 4.183948283277976188 ) ) ;
#3417=CARTESIAN_POINT ( 'NONE',  ( -5.418398423912711870, -0.9480714621563917088, 2.676051716722023244 ) ) ;
#3421=CARTESIAN_POINT ( 'NONE',  ( -4.444597532678119300, -0.7039550926810477227, 1.679999999999999938 ) ) ;
#3424=CARTESIAN_POINT ( 'NONE',  ( 3.119207202478379681, 3.244753828200549695, 6.596051716722022285 ) ) ;
#3432=CARTESIAN_POINT ( 'NONE',  ( 0.9968613283357860011, -5.697241258616382531, 1.976051716722022844 ) ) ;
#3433=CARTESIAN_POINT ( 'NONE',  ( -4.089228379062038066, 4.089228379062021190, 4.900000000000000355 ) ) ;
#3434=CARTESIAN_POINT ( 'NONE',  ( 0.9046671180729951578, -5.711843387010016926, 3.779999999999998472 ) ) ;
#3445=CARTESIAN_POINT ( 'NONE',  ( 3.181980515339458471, 3.181980515339470461, 13.99999999999999822 ) ) ;
#3448=CARTESIAN_POINT ( 'NONE',  ( -0.6479879772514802738, 4.687928535947285091, 1.383948283277976365 ) ) ;
#3453=CARTESIAN_POINT ( 'NONE',  ( -5.152728359536494551, -2.625446233515535077, 4.339999999999999858 ) ) ;
#3456=CARTESIAN_POINT ( 'NONE',  ( -2.496947748567517333, 4.900535883036019058, 10.63999999999999879 ) ) ;
#3460=CARTESIAN_POINT ( 'NONE',  ( -4.940838830814703542, 2.417848759854245078, 14.15605171672202012 ) ) ;
#3464=CARTESIAN_POINT ( 'NONE',  ( 4.258245684917310037, 2.064922774268912686, 1.943948283277976419 ) ) ;
#3467=CARTESIAN_POINT ( 'NONE',  ( 4.940838830814703542, -2.417848759854246410, 4.356051716722023848 ) ) ;
#3472=CARTESIAN_POINT ( 'NONE',  ( 4.673326407553653361, -0.7401821875142525764, 6.019999999999999574 ) ) ;
#3475=CARTESIAN_POINT ( 'NONE',  ( 4.687928535947288644, -0.6479879772514620662, 9.816051716722022036 ) ) ;
#3484=CARTESIAN_POINT ( 'NONE',  ( -5.726445515403654873, 0.8124729078101847746, 2.816051716722022924 ) ) ;
#3485=CARTESIAN_POINT ( 'NONE',  ( 5.711843387010018702, -0.9046671180729751738, 0.4199999999999999289 ) ) ;
#3487=CARTESIAN_POINT ( 'NONE',  ( 5.432285873273257515, 0.8603895577212793411, 11.47999999999999865 ) ) ;
#3500=CARTESIAN_POINT ( 'NONE',  ( -4.458484982038663169, -0.6162731882459353550, 9.083948283277974767 ) ) ;
#3505=CARTESIAN_POINT ( 'NONE',  ( 5.432285873273257515, 0.8603895577212793411, 8.679999999999997939 ) ) ;
#3511=CARTESIAN_POINT ( 'NONE',  ( -0.6162731882459178134, -4.458484982038665834, 2.116051716722023190 ) ) ;
#3513=CARTESIAN_POINT ( 'NONE',  ( 3.244753828200538148, 3.119207202478391672, 13.00394828327797470 ) ) ;
#3516=CARTESIAN_POINT ( 'NONE',  ( -3.826313983664925811, -3.951860609387098489, 7.996051716722022640 ) ) ;
#3521=CARTESIAN_POINT ( 'NONE',  ( -3.181980515339458027, -3.181980515339470905, 9.799999999999998934 ) ) ;
#3522=CARTESIAN_POINT ( 'NONE',  ( 4.049832306626335310, -1.963858260114701215, 7.156051716722023670 ) ) ;
#3531=CARTESIAN_POINT ( 'NONE',  ( 4.155232146225751322, -4.023224611898307934, 4.496051716722022640 ) ) ;
#3533=CARTESIAN_POINT ( 'NONE',  ( 3.889087296526005488, 3.889087296526018811, -3.866961113726609188E-17 ) ) ;
#3534=CARTESIAN_POINT ( 'NONE',  ( -5.152728359536494551, -2.625446233515535077, 12.73999999999999488 ) ) ;
#3548=CARTESIAN_POINT ( 'NONE',  ( 3.244753828200538148, 3.119207202478391672, 13.00394828327797470 ) ) ;
#3553=CARTESIAN_POINT ( 'NONE',  ( -5.711843387010018702, 0.9046671180729746187, 13.01999999999999424 ) ) ;
#3556=CARTESIAN_POINT ( 'NONE',  ( 4.900535883036028828, -2.496947748567499126, 6.159999999999999254 ) ) ;
#3561=CARTESIAN_POINT ( 'NONE',  ( -2.042957248827969252, 4.009529358847651714, 2.239999999999999769 ) ) ;
#3564=CARTESIAN_POINT ( 'NONE',  ( 1.963858260114715870, -4.049832306626327316, 11.04394828327797562 ) ) ;
#3568=CARTESIAN_POINT ( 'NONE',  ( -2.576046737280769605, 4.860232935257343456, 8.836051716722023386 ) ) ;
#3574=CARTESIAN_POINT ( 'NONE',  ( 0.7039550926810297371, 4.444597532678122853, 8.119999999999999218 ) ) ;
#3576=CARTESIAN_POINT ( 'NONE',  ( -0.7039550926810301812, -4.444597532678121965, 3.919999999999999929 ) ) ;
#3586=CARTESIAN_POINT ( 'NONE',  ( -0.8603895577212598011, -5.432285873273260179, 9.519999999999999574 ) ) ;
#3587=CARTESIAN_POINT ( 'NONE',  ( -5.152728359536494551, -2.625446233515535077, 12.73999999999999488 ) ) ;
#3588=CARTESIAN_POINT ( 'NONE',  ( -0.9046671180729963790, 5.711843387010016926, 13.57999999999999474 ) ) ;
#3600=CARTESIAN_POINT ( 'NONE',  ( 2.231261971483764484, 4.173491630687871101, 7.263948283277976259 ) ) ;
#3611=CARTESIAN_POINT ( 'NONE',  ( 4.049832306626335310, -1.963858260114701215, 9.956051716722022604 ) ) ;
#3613=CARTESIAN_POINT ( 'NONE',  ( 0.7916369971161419938, 4.430710083317576320, 12.72394828327797711 ) ) ;
#3621=CIRCLE ( 'NONE', #755, 0.5000000000000000000 ) ;
#3623=CARTESIAN_POINT ( 'NONE',  ( 4.009529358847659708, -2.042957248827953709, 8.959999999999999076 ) ) ;
#3625=CARTESIAN_POINT ( 'NONE',  ( -4.215868657802586128, -2.148092372876348133, 4.339999999999999858 ) ) ;
#3636=CARTESIAN_POINT ( 'NONE',  ( -5.711843387010018702, 0.9046671180729746187, 10.21999999999999709 ) ) ;
#3638=CARTESIAN_POINT ( 'NONE',  ( -2.625446233515515981, -5.152728359536500768, 12.45999999999999552 ) ) ;
#3640=CARTESIAN_POINT ( 'NONE',  ( -3.889087296526005044, -3.889087296526019255, 6.999999999999999112 ) ) ;
#3654=CARTESIAN_POINT ( 'NONE',  ( -3.244753828200538148, -3.119207202478392116, 11.60394828327797434 ) ) ;
#3664=CARTESIAN_POINT ( 'NONE',  ( 3.119207202478379681, 3.244753828200549695, 9.396051716722022107 ) ) ;
#3666=CARTESIAN_POINT ( 'NONE',  ( -5.697241258616385196, 0.9968613283357647958, 3.623948283277976135 ) ) ;
#3674=( BOUNDED_SURFACE ( )  B_SPLINE_SURFACE ( 3, 2, ( 
 ( #3533, #7566, #2592, #3485, #6758, #10020, #1796, #1742, #5024, #4322, #1950, #8268, #1098, #3330, #9005, #7517, #2689, #6708, #5173, #9966, #309, #2745, #151, #4969, #8214, #993, #5908, #5957, #9211, #5806, #9162, #4224, #7466, #8422, #209, #3433, #4121, #7360, #7409, #103, #6556, #1902, #3381, #5121, #948, #9808, #6608, #6656, #2537, #9913, #5756, #9058, #4174, #2642, #5858, #9110, #1846, #5069, #8322, #1051, #4272, #2898, #2003, #4480, #9371, #10069, #7729, #8523, #461, #5224, #1148, #2056, #5282, #6010, #6914, #1255, #2793, #4372, #8472, #411, #6812, #6867, #3688, #1204, #10170, #6119, #9263, #7618, #361, #3638, #10121, #3587, #6060, #4428, #7673, #2843, #9314, #7443, #4355, #9193, #342 ),
 ( #187, #6795, #9895, #1028, #8251, #977, #5105, #5154, #9139, #2672, #5940, #4203, #3417, #8352, #5205, #2775, #6640, #2624, #7498, #5840, #10051, #6691, #6586, #1081, #3467, #9999, #9844, #8451, #9947, #9092, #1827, #2572, #5887, #8299, #8404, #5050, #1182, #134, #4253, #1932, #5005, #1880, #1775, #7595, #4303, #241, #3359, #7550, #293, #9039, #3516, #6735, #2724, #1133, #5787, #5990, #3568, #9247, #1985, #4409, #8099, #3163, #7076, #10329, #1469, #6492, #3110, #4638, #620, #3904, #10388, #2370, #3269, #10497, #9752, #7884, #3848, #830, #4854, #4692, #7935, #5438, #3061, #4013, #6442, #6282, #8782, #2318, #7242, #9538, #4061, #5541, #3213, #1631, #4804, #8676, #1525, #43, #7296, #8728, #2264 ),
 ( #5595, #1412, #5489, #670, #7133, #6333, #8840, #4749, #9590, #7997, #9643, #2427, #726, #3957, #7187, #1582, #10444, #6388, #8049, #780, #9701, #5646, #8891, #198, #4211, #1087, #4311, #5849, #8205, #2679, #1734, #1787, #9100, #4113, #5112, #937, #7454, #9149, #4164, #8359, #3424, #7350, #93, #8995, #3522, #142, #1680, #8155, #7402, #3369, #9903, #300, #7507, #6745, #4907, #889, #7557, #1889, #4959, #6597, #2480, #3322, #1040, #3475, #6546, #5796, #9855, #4261, #9797, #5693, #2580, #248, #8937, #1834, #2526, #9049, #8257, #5745, #9956, #5894, #5014, #2631, #5060, #6647, #6699, #986, #8309, #10214, #1344, #5163, #9201, #400, #10159, #6110, #7822, #553, #2943, #1191, #6961, #8458, #1992 ),
 ( #3729, #8412, #3678, #3781, #6161, #1139, #4417, #2044, #9415, #1939, #5319, #9360, #10005, #4521, #350, #2885, #9254, #1295, #7604, #2735, #5998, #10109, #4362, #5272, #8563, #7659, #7765, #498, #3576, #2148, #2096, #3625, #2833, #5946, #6803, #4572, #6854, #5369, #10059, #2783, #8607, #5211, #6048, #9303, #8511, #1244, #4470, #7716, #451, #6905, #7922, #4624, #7870, #1508, #1568, #5530, #9577, #2356, #605, #3835, #4730, #1618, #9688, #10312, #7062, #3887, #3046, #3202, #3096, #2995, #7982, #10374, #6378, #6211, #4843, #6317, #6265, #9525, #9466, #2306, #4679, #4792, #2251, #8086, #7010, #5474, #5578, #1399, #8769, #8665, #4002, #715, #8713, #10265, #653, #3943, #5423, #7172, #1454, #10429, #7118 ),
 ( #3151, #6426, #9631, #2414, #8825, #8036, #767, #7231, #817, #10486, #2199, #5632, #8878, #8981, #974, #1876, #9089, #5101, #6478, #3255, #9944, #3464, #79, #3308, #8349, #9737, #2621, #5047, #4892, #7390, #922, #5837, #8927, #2668, #4151, #1823, #237, #3414, #4048, #7281, #2468, #5682, #5883, #6688, #6536, #9785, #30, #1666, #8295, #1021, #8142, #131, #3355, #4250, #877, #9135, #6582, #7495, #4103, #6637, #7336, #9840, #2569, #2515, #5728, #1724, #4948, #4200, #7436, #5001, #8192, #5784, #182, #9035, #1771, #8246, #9891, #1981, #1230, #7703, #9400, #2137, #4509, #2771, #8551, #10048, #3564, #6841, #4404, #2031, #4352, #5308, #9993, #5260, #5358, #1283, #2719, #5985, #3613, #7754, #3513 ),
 ( #8399, #9291, #6148, #3715, #7592, #1928, #8448, #335, #488, #7650, #7546, #8499, #388, #440, #290, #1077, #10098, #6792, #1130, #6730, #2824, #9243, #6098, #5202, #4299, #5937, #9189, #6894, #5150, #6037, #1177, #6949, #4456, #3666, #10147, #2872, #9348, #2082, #10203, #2929, #7103, #10302, #8598, #8021, #1556, #7049, #4715, #2342, #10250, #1387, #3872, #6251, #8810, #6412, #2240, #5565, #7809, #2983, #1494, #7157, #702, #9670, #7965, #4778, #3190, #6304, #10361, #7218, #10474, #3930, #3821, #754, #7855, #7909, #10414, #6202, #3987, #3030, #3084, #2401, #9511, #1329, #9563, #9455, #2184, #4612, #4559, #5461, #542, #3768, #8701, #1439, #5516, #6997, #3135, #5408, #8653, #590, #4664, #640, #2292 ),
 ( #9618, #8754, #6364, #2504, #7424, #14, #1011, #5717, #169, #1813, #4986, #9932, #1710, #911, #3244, #2611, #5825, #6466, #2556, #5774, #6572, #4191, #9881, #9024, #9078, #7486, #807, #4830, #6519, #1759, #8233, #3453, #6675, #5038, #7324, #8285, #4091, #8127, #4137, #8966, #9825, #8918, #4241, #4037, #964, #5620, #226, #7267, #67, #8179, #8865, #8076, #3401, #6628, #1606, #9723, #2454, #5668, #1655, #4880, #9776, #3293, #4938, #861, #7376, #120, #3344, #2707, #6720, #8387, #478, #10087, #2761, #5088, #1119, #6831, #10138, #7581, #1865, #8438, #2814, #4342, #1918, #5140, #9281, #1165, #378, #9982, #4393, #325, #2659, #2073, #6084, #3553, #2019, #6885, #4290, #5926, #7639, #6779, #2861 ) ),
 .UNSPECIFIED., .T., .F., .F. ) 
 B_SPLINE_SURFACE_WITH_KNOTS ( ( 4, 3, 4 ),
 ( 3, 2, 2, 2, 2, 2, 2, 2, 2, 2, 2, 2, 2, 2, 2, 2, 2, 2, 2, 2, 2, 2, 2, 2, 2, 2, 2, 2, 2, 2, 2, 2, 2, 2, 2, 2, 2, 2, 2, 2, 2, 2, 2, 2, 2, 2, 2, 2, 2, 2, 3 ),
 ( 0.000000000000000000, 0.5000000000000000000, 1.000000000000000000 ),
 ( 0.000000000000000000, 0.02000000000000000042, 0.04000000000000000083, 0.05999999999999999778, 0.08000000000000000167, 0.1000000000000000056, 0.1199999999999999956, 0.1400000000000000133, 0.1600000000000000033, 0.1799999999999999933, 0.2000000000000000111, 0.2200000000000000011, 0.2399999999999999911, 0.2600000000000000089, 0.2800000000000000266, 0.2999999999999999889, 0.3200000000000000067, 0.3400000000000000244, 0.3599999999999999867, 0.3800000000000000044, 0.4000000000000000222, 0.4199999999999999845, 0.4400000000000000022, 0.4600000000000000200, 0.4799999999999999822, 0.5000000000000000000, 0.5200000000000000178, 0.5400000000000000355, 0.5600000000000000533, 0.5799999999999999600, 0.5999999999999999778, 0.6199999999999999956, 0.6400000000000000133, 0.6600000000000000311, 0.6800000000000000488, 0.6999999999999999556, 0.7199999999999999734, 0.7399999999999999911, 0.7600000000000000089, 0.7800000000000000266, 0.8000000000000000444, 0.8199999999999999512, 0.8399999999999999689, 0.8599999999999999867, 0.8800000000000000044, 0.9000000000000000222, 0.9200000000000000400, 0.9399999999999999467, 0.9599999999999999645, 0.9799999999999999822, 1.000000000000000000 ),
 .UNSPECIFIED. ) 
 GEOMETRIC_REPRESENTATION_ITEM ( )  RATIONAL_B_SPLINE_SURFACE ( (
 ( 1.000000000000000000, 0.9510565162951535312, 1.000000000000000000, 0.9510565162951535312, 1.000000000000000000, 0.9510565162951535312, 1.000000000000000000, 0.9510565162951535312, 1.000000000000000000, 0.9510565162951535312, 1.000000000000000000, 0.9510565162951535312, 1.000000000000000000, 0.9510565162951535312, 1.000000000000000000, 0.9510565162951535312, 1.000000000000000000, 0.9510565162951535312, 1.000000000000000000, 0.9510565162951535312, 1.000000000000000000, 0.9510565162951535312, 1.000000000000000000, 0.9510565162951535312, 1.000000000000000000, 0.9510565162951535312, 1.000000000000000000, 0.9510565162951535312, 1.000000000000000000, 0.9510565162951535312, 1.000000000000000000, 0.9510565162951535312, 1.000000000000000000, 0.9510565162951535312, 1.000000000000000000, 0.9510565162951535312, 1.000000000000000000, 0.9510565162951535312, 1.000000000000000000, 0.9510565162951535312, 1.000000000000000000, 0.9510565162951535312, 1.000000000000000000, 0.9510565162951535312, 1.000000000000000000, 0.9510565162951535312, 1.000000000000000000, 0.9510565162951535312, 1.000000000000000000, 0.9510565162951535312, 1.000000000000000000, 0.9510565162951535312, 1.000000000000000000, 0.9510565162951535312, 1.000000000000000000, 0.9510565162951535312, 1.000000000000000000, 0.9510565162951535312, 1.000000000000000000, 0.9510565162951535312, 1.000000000000000000, 0.9510565162951535312, 1.000000000000000000, 0.9510565162951535312, 1.000000000000000000, 0.9510565162951535312, 1.000000000000000000, 0.9510565162951535312, 1.000000000000000000, 0.9510565162951535312, 1.000000000000000000, 0.9510565162951535312, 1.000000000000000000, 0.9510565162951535312, 1.000000000000000000, 0.9510565162951535312, 1.000000000000000000, 0.9510565162951535312, 1.000000000000000000, 0.9510565162951535312, 1.000000000000000000, 0.9510565162951535312, 1.000000000000000000, 0.9510565162951535312, 1.000000000000000000, 0.9510565162951535312, 1.000000000000000000, 0.9510565162951535312, 1.000000000000000000, 0.9510565162951535312, 1.000000000000000000, 0.9510565162951535312, 1.000000000000000000, 0.9510565162951535312, 1.000000000000000000, 0.9510565162951535312, 1.000000000000000000, 0.9510565162951535312, 1.000000000000000000, 0.9510565162951535312, 1.000000000000000000),
 ( 0.3333333333333333703, 0.3170188387650512141, 0.3333333333333333703, 0.3170188387650512141, 0.3333333333333333703, 0.3170188387650512141, 0.3333333333333333703, 0.3170188387650512141, 0.3333333333333333703, 0.3170188387650512141, 0.3333333333333333703, 0.3170188387650512141, 0.3333333333333333703, 0.3170188387650512141, 0.3333333333333333703, 0.3170188387650512141, 0.3333333333333333703, 0.3170188387650512141, 0.3333333333333333703, 0.3170188387650512141, 0.3333333333333333703, 0.3170188387650512141, 0.3333333333333333703, 0.3170188387650512141, 0.3333333333333333703, 0.3170188387650512141, 0.3333333333333333703, 0.3170188387650512141, 0.3333333333333333703, 0.3170188387650512141, 0.3333333333333333703, 0.3170188387650512141, 0.3333333333333333703, 0.3170188387650512141, 0.3333333333333333703, 0.3170188387650512141, 0.3333333333333333703, 0.3170188387650512141, 0.3333333333333333703, 0.3170188387650512141, 0.3333333333333333703, 0.3170188387650512141, 0.3333333333333333703, 0.3170188387650512141, 0.3333333333333333703, 0.3170188387650512141, 0.3333333333333333703, 0.3170188387650512141, 0.3333333333333333703, 0.3170188387650512141, 0.3333333333333333703, 0.3170188387650512141, 0.3333333333333333703, 0.3170188387650512141, 0.3333333333333333703, 0.3170188387650512141, 0.3333333333333333703, 0.3170188387650512141, 0.3333333333333333703, 0.3170188387650512141, 0.3333333333333333703, 0.3170188387650512141, 0.3333333333333333703, 0.3170188387650512141, 0.3333333333333333703, 0.3170188387650512141, 0.3333333333333333703, 0.3170188387650512141, 0.3333333333333333703, 0.3170188387650512141, 0.3333333333333333703, 0.3170188387650512141, 0.3333333333333333703, 0.3170188387650512141, 0.3333333333333333703, 0.3170188387650512141, 0.3333333333333333703, 0.3170188387650512141, 0.3333333333333333703, 0.3170188387650512141, 0.3333333333333333703, 0.3170188387650512141, 0.3333333333333333703, 0.3170188387650512141, 0.3333333333333333703, 0.3170188387650512141, 0.3333333333333333703, 0.3170188387650512141, 0.3333333333333333703, 0.3170188387650512141, 0.3333333333333333703, 0.3170188387650512141, 0.3333333333333333703, 0.3170188387650512141, 0.3333333333333333703, 0.3170188387650512141, 0.3333333333333333703, 0.3170188387650512141, 0.3333333333333333703, 0.3170188387650512141, 0.3333333333333333703),
 ( 0.3333333333333333703, 0.3170188387650512141, 0.3333333333333333703, 0.3170188387650512141, 0.3333333333333333703, 0.3170188387650512141, 0.3333333333333333703, 0.3170188387650512141, 0.3333333333333333703, 0.3170188387650512141, 0.3333333333333333703, 0.3170188387650512141, 0.3333333333333333703, 0.3170188387650512141, 0.3333333333333333703, 0.3170188387650512141, 0.3333333333333333703, 0.3170188387650512141, 0.3333333333333333703, 0.3170188387650512141, 0.3333333333333333703, 0.3170188387650512141, 0.3333333333333333703, 0.3170188387650512141, 0.3333333333333333703, 0.3170188387650512141, 0.3333333333333333703, 0.3170188387650512141, 0.3333333333333333703, 0.3170188387650512141, 0.3333333333333333703, 0.3170188387650512141, 0.3333333333333333703, 0.3170188387650512141, 0.3333333333333333703, 0.3170188387650512141, 0.3333333333333333703, 0.3170188387650512141, 0.3333333333333333703, 0.3170188387650512141, 0.3333333333333333703, 0.3170188387650512141, 0.3333333333333333703, 0.3170188387650512141, 0.3333333333333333703, 0.3170188387650512141, 0.3333333333333333703, 0.3170188387650512141, 0.3333333333333333703, 0.3170188387650512141, 0.3333333333333333703, 0.3170188387650512141, 0.3333333333333333703, 0.3170188387650512141, 0.3333333333333333703, 0.3170188387650512141, 0.3333333333333333703, 0.3170188387650512141, 0.3333333333333333703, 0.3170188387650512141, 0.3333333333333333703, 0.3170188387650512141, 0.3333333333333333703, 0.3170188387650512141, 0.3333333333333333703, 0.3170188387650512141, 0.3333333333333333703, 0.3170188387650512141, 0.3333333333333333703, 0.3170188387650512141, 0.3333333333333333703, 0.3170188387650512141, 0.3333333333333333703, 0.3170188387650512141, 0.3333333333333333703, 0.3170188387650512141, 0.3333333333333333703, 0.3170188387650512141, 0.3333333333333333703, 0.3170188387650512141, 0.3333333333333333703, 0.3170188387650512141, 0.3333333333333333703, 0.3170188387650512141, 0.3333333333333333703, 0.3170188387650512141, 0.3333333333333333703, 0.3170188387650512141, 0.3333333333333333703, 0.3170188387650512141, 0.3333333333333333703, 0.3170188387650512141, 0.3333333333333333703, 0.3170188387650512141, 0.3333333333333333703, 0.3170188387650512141, 0.3333333333333333703, 0.3170188387650512141, 0.3333333333333333703, 0.3170188387650512141, 0.3333333333333333703),
 ( 1.000000000000000000, 0.9510565162951535312, 1.000000000000000000, 0.9510565162951535312, 1.000000000000000000, 0.9510565162951535312, 1.000000000000000000, 0.9510565162951535312, 1.000000000000000000, 0.9510565162951535312, 1.000000000000000000, 0.9510565162951535312, 1.000000000000000000, 0.9510565162951535312, 1.000000000000000000, 0.9510565162951535312, 1.000000000000000000, 0.9510565162951535312, 1.000000000000000000, 0.9510565162951535312, 1.000000000000000000, 0.9510565162951535312, 1.000000000000000000, 0.9510565162951535312, 1.000000000000000000, 0.9510565162951535312, 1.000000000000000000, 0.9510565162951535312, 1.000000000000000000, 0.9510565162951535312, 1.000000000000000000, 0.9510565162951535312, 1.000000000000000000, 0.9510565162951535312, 1.000000000000000000, 0.9510565162951535312, 1.000000000000000000, 0.9510565162951535312, 1.000000000000000000, 0.9510565162951535312, 1.000000000000000000, 0.9510565162951535312, 1.000000000000000000, 0.9510565162951535312, 1.000000000000000000, 0.9510565162951535312, 1.000000000000000000, 0.9510565162951535312, 1.000000000000000000, 0.9510565162951535312, 1.000000000000000000, 0.9510565162951535312, 1.000000000000000000, 0.9510565162951535312, 1.000000000000000000, 0.9510565162951535312, 1.000000000000000000, 0.9510565162951535312, 1.000000000000000000, 0.9510565162951535312, 1.000000000000000000, 0.9510565162951535312, 1.000000000000000000, 0.9510565162951535312, 1.000000000000000000, 0.9510565162951535312, 1.000000000000000000, 0.9510565162951535312, 1.000000000000000000, 0.9510565162951535312, 1.000000000000000000, 0.9510565162951535312, 1.000000000000000000, 0.9510565162951535312, 1.000000000000000000, 0.9510565162951535312, 1.000000000000000000, 0.9510565162951535312, 1.000000000000000000, 0.9510565162951535312, 1.000000000000000000, 0.9510565162951535312, 1.000000000000000000, 0.9510565162951535312, 1.000000000000000000, 0.9510565162951535312, 1.000000000000000000, 0.9510565162951535312, 1.000000000000000000, 0.9510565162951535312, 1.000000000000000000, 0.9510565162951535312, 1.000000000000000000, 0.9510565162951535312, 1.000000000000000000, 0.9510565162951535312, 1.000000000000000000, 0.9510565162951535312, 1.000000000000000000, 0.9510565162951535312, 1.000000000000000000),
 ( 0.3333333333333333703, 0.3170188387650512141, 0.3333333333333333703, 0.3170188387650512141, 0.3333333333333333703, 0.3170188387650512141, 0.3333333333333333703, 0.3170188387650512141, 0.3333333333333333703, 0.3170188387650512141, 0.3333333333333333703, 0.3170188387650512141, 0.3333333333333333703, 0.3170188387650512141, 0.3333333333333333703, 0.3170188387650512141, 0.3333333333333333703, 0.3170188387650512141, 0.3333333333333333703, 0.3170188387650512141, 0.3333333333333333703, 0.3170188387650512141, 0.3333333333333333703, 0.3170188387650512141, 0.3333333333333333703, 0.3170188387650512141, 0.3333333333333333703, 0.3170188387650512141, 0.3333333333333333703, 0.3170188387650512141, 0.3333333333333333703, 0.3170188387650512141, 0.3333333333333333703, 0.3170188387650512141, 0.3333333333333333703, 0.3170188387650512141, 0.3333333333333333703, 0.3170188387650512141, 0.3333333333333333703, 0.3170188387650512141, 0.3333333333333333703, 0.3170188387650512141, 0.3333333333333333703, 0.3170188387650512141, 0.3333333333333333703, 0.3170188387650512141, 0.3333333333333333703, 0.3170188387650512141, 0.3333333333333333703, 0.3170188387650512141, 0.3333333333333333703, 0.3170188387650512141, 0.3333333333333333703, 0.3170188387650512141, 0.3333333333333333703, 0.3170188387650512141, 0.3333333333333333703, 0.3170188387650512141, 0.3333333333333333703, 0.3170188387650512141, 0.3333333333333333703, 0.3170188387650512141, 0.3333333333333333703, 0.3170188387650512141, 0.3333333333333333703, 0.3170188387650512141, 0.3333333333333333703, 0.3170188387650512141, 0.3333333333333333703, 0.3170188387650512141, 0.3333333333333333703, 0.3170188387650512141, 0.3333333333333333703, 0.3170188387650512141, 0.3333333333333333703, 0.3170188387650512141, 0.3333333333333333703, 0.3170188387650512141, 0.3333333333333333703, 0.3170188387650512141, 0.3333333333333333703, 0.3170188387650512141, 0.3333333333333333703, 0.3170188387650512141, 0.3333333333333333703, 0.3170188387650512141, 0.3333333333333333703, 0.3170188387650512141, 0.3333333333333333703, 0.3170188387650512141, 0.3333333333333333703, 0.3170188387650512141, 0.3333333333333333703, 0.3170188387650512141, 0.3333333333333333703, 0.3170188387650512141, 0.3333333333333333703, 0.3170188387650512141, 0.3333333333333333703, 0.3170188387650512141, 0.3333333333333333703),
 ( 0.3333333333333333703, 0.3170188387650512141, 0.3333333333333333703, 0.3170188387650512141, 0.3333333333333333703, 0.3170188387650512141, 0.3333333333333333703, 0.3170188387650512141, 0.3333333333333333703, 0.3170188387650512141, 0.3333333333333333703, 0.3170188387650512141, 0.3333333333333333703, 0.3170188387650512141, 0.3333333333333333703, 0.3170188387650512141, 0.3333333333333333703, 0.3170188387650512141, 0.3333333333333333703, 0.3170188387650512141, 0.3333333333333333703, 0.3170188387650512141, 0.3333333333333333703, 0.3170188387650512141, 0.3333333333333333703, 0.3170188387650512141, 0.3333333333333333703, 0.3170188387650512141, 0.3333333333333333703, 0.3170188387650512141, 0.3333333333333333703, 0.3170188387650512141, 0.3333333333333333703, 0.3170188387650512141, 0.3333333333333333703, 0.3170188387650512141, 0.3333333333333333703, 0.3170188387650512141, 0.3333333333333333703, 0.3170188387650512141, 0.3333333333333333703, 0.3170188387650512141, 0.3333333333333333703, 0.3170188387650512141, 0.3333333333333333703, 0.3170188387650512141, 0.3333333333333333703, 0.3170188387650512141, 0.3333333333333333703, 0.3170188387650512141, 0.3333333333333333703, 0.3170188387650512141, 0.3333333333333333703, 0.3170188387650512141, 0.3333333333333333703, 0.3170188387650512141, 0.3333333333333333703, 0.3170188387650512141, 0.3333333333333333703, 0.3170188387650512141, 0.3333333333333333703, 0.3170188387650512141, 0.3333333333333333703, 0.3170188387650512141, 0.3333333333333333703, 0.3170188387650512141, 0.3333333333333333703, 0.3170188387650512141, 0.3333333333333333703, 0.3170188387650512141, 0.3333333333333333703, 0.3170188387650512141, 0.3333333333333333703, 0.3170188387650512141, 0.3333333333333333703, 0.3170188387650512141, 0.3333333333333333703, 0.3170188387650512141, 0.3333333333333333703, 0.3170188387650512141, 0.3333333333333333703, 0.3170188387650512141, 0.3333333333333333703, 0.3170188387650512141, 0.3333333333333333703, 0.3170188387650512141, 0.3333333333333333703, 0.3170188387650512141, 0.3333333333333333703, 0.3170188387650512141, 0.3333333333333333703, 0.3170188387650512141, 0.3333333333333333703, 0.3170188387650512141, 0.3333333333333333703, 0.3170188387650512141, 0.3333333333333333703, 0.3170188387650512141, 0.3333333333333333703, 0.3170188387650512141, 0.3333333333333333703),
 ( 1.000000000000000000, 0.9510565162951535312, 1.000000000000000000, 0.9510565162951535312, 1.000000000000000000, 0.9510565162951535312, 1.000000000000000000, 0.9510565162951535312, 1.000000000000000000, 0.9510565162951535312, 1.000000000000000000, 0.9510565162951535312, 1.000000000000000000, 0.9510565162951535312, 1.000000000000000000, 0.9510565162951535312, 1.000000000000000000, 0.9510565162951535312, 1.000000000000000000, 0.9510565162951535312, 1.000000000000000000, 0.9510565162951535312, 1.000000000000000000, 0.9510565162951535312, 1.000000000000000000, 0.9510565162951535312, 1.000000000000000000, 0.9510565162951535312, 1.000000000000000000, 0.9510565162951535312, 1.000000000000000000, 0.9510565162951535312, 1.000000000000000000, 0.9510565162951535312, 1.000000000000000000, 0.9510565162951535312, 1.000000000000000000, 0.9510565162951535312, 1.000000000000000000, 0.9510565162951535312, 1.000000000000000000, 0.9510565162951535312, 1.000000000000000000, 0.9510565162951535312, 1.000000000000000000, 0.9510565162951535312, 1.000000000000000000, 0.9510565162951535312, 1.000000000000000000, 0.9510565162951535312, 1.000000000000000000, 0.9510565162951535312, 1.000000000000000000, 0.9510565162951535312, 1.000000000000000000, 0.9510565162951535312, 1.000000000000000000, 0.9510565162951535312, 1.000000000000000000, 0.9510565162951535312, 1.000000000000000000, 0.9510565162951535312, 1.000000000000000000, 0.9510565162951535312, 1.000000000000000000, 0.9510565162951535312, 1.000000000000000000, 0.9510565162951535312, 1.000000000000000000, 0.9510565162951535312, 1.000000000000000000, 0.9510565162951535312, 1.000000000000000000, 0.9510565162951535312, 1.000000000000000000, 0.9510565162951535312, 1.000000000000000000, 0.9510565162951535312, 1.000000000000000000, 0.9510565162951535312, 1.000000000000000000, 0.9510565162951535312, 1.000000000000000000, 0.9510565162951535312, 1.000000000000000000, 0.9510565162951535312, 1.000000000000000000, 0.9510565162951535312, 1.000000000000000000, 0.9510565162951535312, 1.000000000000000000, 0.9510565162951535312, 1.000000000000000000, 0.9510565162951535312, 1.000000000000000000, 0.9510565162951535312, 1.000000000000000000, 0.9510565162951535312, 1.000000000000000000, 0.9510565162951535312, 1.000000000000000000) ) ) 
 REPRESENTATION_ITEM ( '' )  SURFACE ( )  );
#3675=CARTESIAN_POINT ( 'NONE',  ( -4.009529358847660596, 2.042957248827953265, 13.15999999999999837 ) ) ;
#3678=CARTESIAN_POINT ( 'NONE',  ( 4.444597532678119300, 0.7039550926810472786, 0.2799999999999999711 ) ) ;
#3687=CARTESIAN_POINT ( 'NONE',  ( 5.110351332421769754, 2.708615832122969191, 9.536051716722020899 ) ) ;
#3688=CARTESIAN_POINT ( 'NONE',  ( 5.432285873273257515, 0.8603895577212793411, 11.47999999999999865 ) ) ;
#3689=CARTESIAN_POINT ( 'NONE',  ( -4.089228379062038066, 4.089228379062021190, 10.50000000000000000 ) ) ;
#3699=CARTESIAN_POINT ( 'NONE',  ( -4.458484982038663169, -0.6162731882459353550, 11.88394828327797548 ) ) ;
#3712=CARTESIAN_POINT ( 'NONE',  ( 2.122056237541221524, -3.969226411068978777, 13.03605171672202090 ) ) ;
#3715=CARTESIAN_POINT ( 'NONE',  ( 5.697241258616385196, -0.9968613283357656840, -0.5760517167220230439 ) ) ;
#3729=CARTESIAN_POINT ( 'NONE',  ( 3.181980515339458471, 3.181980515339470461, 2.232096619617652273E-17 ) ) ;
#3739=CARTESIAN_POINT ( 'NONE',  ( 4.940838830814703542, -2.417848759854246410, 7.156051716722023670 ) ) ;
#3752=CARTESIAN_POINT ( 'NONE',  ( -0.8124729078102072011, 5.726445515403652209, 6.983948283277976010 ) ) ;
#3764=CARTESIAN_POINT ( 'NONE',  ( 3.345732310141667387, -3.345732310141653620, 9.099999999999999645 ) ) ;
#3768=CARTESIAN_POINT ( 'NONE',  ( -2.708615832122950096, -5.110351332421780413, 11.46394828327797555 ) ) ;
#3781=CARTESIAN_POINT ( 'NONE',  ( 4.673326407553653361, -0.7401821875142523544, 0.4199999999999999845 ) ) ;
#3789=CARTESIAN_POINT ( 'NONE',  ( 4.940838830814703542, -2.417848759854246410, 12.75605171672202331 ) ) ;
#3803=CARTESIAN_POINT ( 'NONE',  ( -5.195105386651219348, -2.542276634908102295, 0.5439482832779766186 ) ) ;
#3818=CARTESIAN_POINT ( 'NONE',  ( 4.673326407553653361, -0.7401821875142523544, 6.019999999999999574 ) ) ;
#3821=CARTESIAN_POINT ( 'NONE',  ( -3.951860609387083834, -3.826313983664940466, 8.803948283277977183 ) ) ;
#3835=CARTESIAN_POINT ( 'NONE',  ( 2.148092372876330369, 4.215868657802593233, 8.259999999999999787 ) ) ;
#3843=CARTESIAN_POINT ( 'NONE',  ( -3.826313983664925811, -3.951860609387098489, 13.59605171672202140 ) ) ;
#3848=CARTESIAN_POINT ( 'NONE',  ( -2.576046737280769605, 4.860232935257343456, 11.63605171672202232 ) ) ;
#3856=FACE_OUTER_BOUND ( 'NONE', #10349, .T. ) ;
#3858=CARTESIAN_POINT ( 'NONE',  ( -2.708615832122950096, -5.110351332421780413, 3.063948283277976081 ) ) ;
#3868=CARTESIAN_POINT ( 'NONE',  ( 2.042957248827968808, -4.009529358847652603, 3.639999999999999680 ) ) ;
#3872=CARTESIAN_POINT ( 'NONE',  ( -3.951860609387083834, -3.826313983664940466, 6.003948283277975584 ) ) ;
#3876=CIRCLE ( 'NONE', #6238, 0.5000000000000000000 ) ;
#3887=CARTESIAN_POINT ( 'NONE',  ( 3.345732310141667387, -3.345732310141653620, 9.099999999999999645 ) ) ;
#3888=UNCERTAINTY_MEASURE_WITH_UNIT (LENGTH_MEASURE( 1.000000000000000082E-05 ), #10391, 'distance_accuracy_value', 'NONE');
#3897=CARTESIAN_POINT ( 'NONE',  ( 0.7727076532861471003, 5.446173322633805824, 11.91605171672202346 ) ) ;
#3904=CARTESIAN_POINT ( 'NONE',  ( -2.542276634908081423, -5.195105386651227342, 10.65605171672202012 ) ) ;
#3907=( NAMED_UNIT ( * ) PLANE_ANGLE_UNIT ( ) SI_UNIT ( $, .RADIAN. ) );
#3915=CARTESIAN_POINT ( 'NONE',  ( 2.708615832122949652, 5.110351332421781301, 4.463948283277976437 ) ) ;
#3928=CARTESIAN_POINT ( 'NONE',  ( -4.444597532678119300, -0.7039550926810477227, 7.279999999999999361 ) ) ;
#3930=CARTESIAN_POINT ( 'NONE',  ( -2.708615832122950096, -5.110351332421780413, 8.663948283277974838 ) ) ;
#3943=CARTESIAN_POINT ( 'NONE',  ( -3.345732310141667831, 3.345732310141653620, 13.29999999999999538 ) ) ;
#3957=CARTESIAN_POINT ( 'NONE',  ( -4.687928535947287756, 0.6479879772514611780, 2.816051716722022924 ) ) ;
#3967=CARTESIAN_POINT ( 'NONE',  ( -2.625446233515515981, -5.152728359536500768, 6.859999999999999432 ) ) ;
#3969=CARTESIAN_POINT ( 'NONE',  ( 2.708615832122949652, 5.110351332421781301, 1.663948283277976392 ) ) ;
#3984=CARTESIAN_POINT ( 'NONE',  ( -4.215868657802586128, -2.148092372876348133, 4.339999999999999858 ) ) ;
#3987=CARTESIAN_POINT ( 'NONE',  ( -2.417848759854264618, 4.940838830814694660, 9.643948283277975264 ) ) ;
#3992=CARTESIAN_POINT ( 'NONE',  ( 5.711843387010019590, -0.9046671180729753958, 0.4199999999999999289 ) ) ;
#4002=CARTESIAN_POINT ( 'NONE',  ( -3.181980515339458027, -3.181980515339470905, 12.59999999999999787 ) ) ;
#4008=CARTESIAN_POINT ( 'NONE',  ( 3.889087296526005488, 3.889087296526018811, 13.99999999999999822 ) ) ;
#4011=CARTESIAN_POINT ( 'NONE',  ( -2.042957248827969252, 4.009529358847651714, 2.239999999999999769 ) ) ;
#4013=CARTESIAN_POINT ( 'NONE',  ( 5.726445515403654873, -0.8124729078101852187, 12.61605171672202097 ) ) ;
#4020=CARTESIAN_POINT ( 'NONE',  ( 2.496947748567516889, -4.900535883036019946, 6.439999999999999503 ) ) ;
#4022=CARTESIAN_POINT ( 'NONE',  ( 2.625446233515515537, 5.152728359536502545, 2.659999999999998366 ) ) ;
#4032=CARTESIAN_POINT ( 'NONE',  ( -0.6479879772514802738, 4.687928535947285091, 4.183948283277976188 ) ) ;
#4037=CARTESIAN_POINT ( 'NONE',  ( 5.711843387010018702, -0.9046671180729751738, 6.019999999999999574 ) ) ;
#4040=CARTESIAN_POINT ( 'NONE',  ( 2.625446233515515093, 5.152728359536503433, 2.659999999999999254 ) ) ;
#4048=CARTESIAN_POINT ( 'NONE',  ( 0.7916369971161419938, 4.430710083317576320, 4.323948283277975868 ) ) ;
#4056=CARTESIAN_POINT ( 'NONE',  ( 3.345732310141667387, -3.345732310141654064, 3.499999999999999112 ) ) ;
#4061=CARTESIAN_POINT ( 'NONE',  ( -3.826313983664925811, -3.951860609387098489, 13.59605171672202140 ) ) ;
#4070=CARTESIAN_POINT ( 'NONE',  ( -0.9046671180729963790, 5.711843387010016926, 7.979999999999999538 ) ) ;
#4072=CARTESIAN_POINT ( 'NONE',  ( 0.9480714621563713917, 5.418398423912717199, 9.923948283277976401 ) ) ;
#4087=CARTESIAN_POINT ( 'NONE',  ( -3.345732310141667831, 3.345732310141653620, 13.29999999999999538 ) ) ;
#4091=CARTESIAN_POINT ( 'NONE',  ( -2.496947748567517333, 4.900535883036019058, 5.039999999999999147 ) ) ;
#4100=CARTESIAN_POINT ( 'NONE',  ( -4.173491630687863108, -2.231261971483782691, 8.136051716722024096 ) ) ;
#4103=CARTESIAN_POINT ( 'NONE',  ( 0.7916369971161419938, 4.430710083317576320, 7.123948283277974802 ) ) ;
#4111=CARTESIAN_POINT ( 'NONE',  ( 3.345732310141667387, -3.345732310141654064, 0.6999999999999997335 ) ) ;
#4113=CARTESIAN_POINT ( 'NONE',  ( -4.687928535947287756, 0.6479879772514611780, 5.616051716722022746 ) ) ;
#4117=DIRECTION ( 'NONE',  ( 0.7071067811865467956, 0.7071067811865484609, -6.099057733344262077E-17 ) ) ;
#4120=CARTESIAN_POINT ( 'NONE',  ( -3.889087296526005044, -3.889087296526019255, 1.399999999999999689 ) ) ;
#4121=CARTESIAN_POINT ( 'NONE',  ( -2.496947748567517333, 4.900535883036019058, 5.039999999999999147 ) ) ;
#4122=CARTESIAN_POINT ( 'NONE',  ( -2.625446233515515981, -5.152728359536500768, 1.259999999999999787 ) ) ;
#4134=CARTESIAN_POINT ( 'NONE',  ( -3.181980515339458027, -3.181980515339470905, 12.59999999999999787 ) ) ;
#4137=CARTESIAN_POINT ( 'NONE',  ( 0.8603895577212593571, 5.432285873273261068, 5.319999999999999396 ) ) ;
#4138=( GEOMETRIC_REPRESENTATION_CONTEXT ( 3 ) GLOBAL_UNCERTAINTY_ASSIGNED_CONTEXT ( ( #10375 ) ) GLOBAL_UNIT_ASSIGNED_CONTEXT ( ( #9434, #3907, #6336 ) ) REPRESENTATION_CONTEXT ( 'NONE', 'WORKASPACE' ) );
#4141=CARTESIAN_POINT ( 'NONE',  ( 2.496947748567516889, -4.900535883036019946, 3.639999999999999680 ) ) ;
#4148=CARTESIAN_POINT ( 'NONE',  ( -3.411736077305382420, 3.279728542977939476, 3.096051716722023617 ) ) ;
#4149=DIRECTION ( 'NONE',  ( 0.7043149233066460235, -0.7043149233066438031, 0.08877487040322794287 ) ) ;
#4151=CARTESIAN_POINT ( 'NONE',  ( -3.969226411068985882, 2.122056237541205537, 3.763948283277976703 ) ) ;
#4154=ADVANCED_FACE ( 'NONE', ( #4335 ), #1062, .F. ) ;
#4164=CARTESIAN_POINT ( 'NONE',  ( 0.6162731882459174804, 4.458484982038668498, 6.316051716722022924 ) ) ;
#4173=CARTESIAN_POINT ( 'NONE',  ( 5.432285873273257515, 0.8603895577212793411, 5.879999999999999893 ) ) ;
#4174=CARTESIAN_POINT ( 'NONE',  ( -5.432285873273256627, -0.8603895577212797852, 7.279999999999999361 ) ) ;
#4175=CARTESIAN_POINT ( 'NONE',  ( -3.889087296526005044, -3.889087296526019255, 4.200000000000000178 ) ) ;
#4187=CARTESIAN_POINT ( 'NONE',  ( 4.458484982038663169, 0.6162731882459350219, 4.883948283277976365 ) ) ;
#4191=CARTESIAN_POINT ( 'NONE',  ( 5.152728359536493663, 2.625446233515533745, 2.939999999999999059 ) ) ;
#4193=CARTESIAN_POINT ( 'NONE',  ( -2.496947748567517333, 4.900535883036019058, 5.039999999999999147 ) ) ;
#4197=CARTESIAN_POINT ( 'NONE',  ( 2.122056237541221524, -3.969226411068978777, 7.436051716722023031 ) ) ;
#4200=CARTESIAN_POINT ( 'NONE',  ( 0.6479879772514793856, -4.687928535947285091, 8.383948283277975477 ) ) ;
#4203=CARTESIAN_POINT ( 'NONE',  ( -5.110351332421769754, -2.708615832122969191, 2.536051716722023119 ) ) ;
#4211=CARTESIAN_POINT ( 'NONE',  ( 4.049832306626335310, -1.963858260114701215, 4.356051716722023848 ) ) ;
#4221=AXIS2_PLACEMENT_3D ( 'NONE', #3445, #5133, #10033 ) ;
#4222=CARTESIAN_POINT ( 'NONE',  ( -2.496947748567517333, 4.900535883036019058, 13.43999999999999950 ) ) ;
#4224=CARTESIAN_POINT ( 'NONE',  ( -5.152728359536494551, -2.625446233515535077, 4.339999999999999858 ) ) ;
#4225=CARTESIAN_POINT ( 'NONE',  ( 4.089228379062037178, -4.089228379062022967, 3.499999999999998668 ) ) ;
#4235=STYLED_ITEM ( 'NONE', ( #8670 ), #8241 ) ;
#4237=CARTESIAN_POINT ( 'NONE',  ( -0.7039550926810301812, -4.444597532678121965, 12.31999999999999851 ) ) ;
#4241=CARTESIAN_POINT ( 'NONE',  ( 5.432285873273257515, 0.8603895577212793411, 5.879999999999999893 ) ) ;
#4243=CARTESIAN_POINT ( 'NONE',  ( -0.8603895577212598011, -5.432285873273260179, 9.519999999999999574 ) ) ;
#4248=CARTESIAN_POINT ( 'NONE',  ( 0.6162731882459174804, 4.458484982038668498, 3.516051716722023102 ) ) ;
#4250=CARTESIAN_POINT ( 'NONE',  ( -4.658724279160018078, 0.8323763977770419764, 6.423948283277978177 ) ) ;
#4253=CARTESIAN_POINT ( 'NONE',  ( 0.7727076532861471003, 5.446173322633805824, 6.316051716722022924 ) ) ;
#4258=CARTESIAN_POINT ( 'NONE',  ( -2.042957248827969252, 4.009529358847651714, 10.63999999999999879 ) ) ;
#4261=CARTESIAN_POINT ( 'NONE',  ( 0.8323763977770604061, -4.658724279160015413, 10.37605171672202253 ) ) ;
#4271=CARTESIAN_POINT ( 'NONE',  ( 4.089228379062037178, -4.089228379062022967, 9.099999999999999645 ) ) ;
#4272=CARTESIAN_POINT ( 'NONE',  ( 3.889087296526005488, 3.889087296526018811, 8.400000000000000355 ) ) ;
#4273=CARTESIAN_POINT ( 'NONE',  ( -3.889087296526005044, -3.889087296526019255, 9.799999999999998934 ) ) ;
#4287=CARTESIAN_POINT ( 'NONE',  ( -4.658724279160018078, 0.8323763977770419764, 12.02394828327797427 ) ) ;
#4290=CARTESIAN_POINT ( 'NONE',  ( -2.496947748567517333, 4.900535883036019058, 13.43999999999999950 ) ) ;
#4293=CARTESIAN_POINT ( 'NONE',  ( -4.089228379062038066, 4.089228379062022078, 10.50000000000000000 ) ) ;
#4297=CARTESIAN_POINT ( 'NONE',  ( 0.6162731882459174804, 4.458484982038668498, 6.316051716722022924 ) ) ;
#4299=CARTESIAN_POINT ( 'NONE',  ( 4.860232935257354114, -2.576046737280751842, 2.363948283277975904 ) ) ;
#4303=CARTESIAN_POINT ( 'NONE',  ( 4.940838830814703542, -2.417848759854246410, 7.156051716722023670 ) ) ;
#4309=CARTESIAN_POINT ( 'NONE',  ( 4.009529358847659708, -2.042957248827953709, 6.159999999999999254 ) ) ;
#4311=CARTESIAN_POINT ( 'NONE',  ( 2.122056237541221524, -3.969226411068978777, 4.636051716722022320 ) ) ;
#4321=CARTESIAN_POINT ( 'NONE',  ( 5.726445515403654873, -0.8124729078101852187, 1.416051716722023235 ) ) ;
#4322=CARTESIAN_POINT ( 'NONE',  ( -2.625446233515515981, -5.152728359536500768, 1.259999999999999787 ) ) ;
#4323=CARTESIAN_POINT ( 'NONE',  ( -5.711843387010018702, 0.9046671180729746187, 10.21999999999999709 ) ) ;
#4335=FACE_OUTER_BOUND ( 'NONE', #4369, .T. ) ;
#4338=CARTESIAN_POINT ( 'NONE',  ( 0.7916369971161419938, 4.430710083317576320, 12.72394828327797711 ) ) ;
#4342=CARTESIAN_POINT ( 'NONE',  ( 5.152728359536493663, 2.625446233515533745, 11.33999999999999808 ) ) ;
#4344=CARTESIAN_POINT ( 'NONE',  ( -4.089228379062038066, 4.089228379062022078, 7.699999999999998401 ) ) ;
#4348=CARTESIAN_POINT ( 'NONE',  ( -4.009529358847660596, 2.042957248827953265, 1.959999999999999964 ) ) ;
#4352=CARTESIAN_POINT ( 'NONE',  ( -3.244753828200538148, -3.119207202478392116, 11.60394828327797434 ) ) ;
#4355=CARTESIAN_POINT ( 'NONE',  ( 0.8603895577212593571, 5.432285873273261068, 13.71999999999999886 ) ) ;
#4360=CARTESIAN_POINT ( 'NONE',  ( 4.444597532678119300, 0.7039550926810472786, 5.879999999999999893 ) ) ;
#4362=CARTESIAN_POINT ( 'NONE',  ( 4.444597532678119300, 0.7039550926810472786, 3.079999999999999627 ) ) ;
#4369=EDGE_LOOP ( 'NONE', ( #2120, #9924 ) ) ;
#4370=CARTESIAN_POINT ( 'NONE',  ( 2.625446233515515537, 5.152728359536502545, 13.85999999999999766 ) ) ;
#4372=CARTESIAN_POINT ( 'NONE',  ( -0.9046671180729963790, 5.711843387010016926, 10.77999999999999936 ) ) ;
#4373=CARTESIAN_POINT ( 'NONE',  ( -4.089228379062038066, 4.089228379062021190, 13.29999999999999538 ) ) ;
#4376=ADVANCED_FACE ( 'NONE', ( #3856 ), #5413, .T. ) ;
#4388=CARTESIAN_POINT ( 'NONE',  ( 0.7916369971161419938, 4.430710083317576320, 7.123948283277974802 ) ) ;
#4393=CARTESIAN_POINT ( 'NONE',  ( -0.8603895577212598011, -5.432285873273260179, 12.31999999999999851 ) ) ;
#4395=CARTESIAN_POINT ( 'NONE',  ( 2.625446233515515093, 5.152728359536503433, 13.85999999999999943 ) ) ;
#4402=CARTESIAN_POINT ( 'NONE',  ( 2.064922774268895811, 4.258245684917319807, 12.05605171672202047 ) ) ;
#4404=CARTESIAN_POINT ( 'NONE',  ( -0.7916369971161423269, -4.430710083317576320, 11.32394828327797676 ) ) ;
#4409=CARTESIAN_POINT ( 'NONE',  ( 2.542276634908080535, 5.195105386651229118, 9.256051716722023315 ) ) ;
#4415=CARTESIAN_POINT ( 'NONE',  ( 4.215868657802586128, 2.148092372876346801, 11.33999999999999808 ) ) ;
#4417=CARTESIAN_POINT ( 'NONE',  ( 2.042957248827968808, -4.009529358847652603, 0.8399999999999999689 ) ) ;
#4427=CARTESIAN_POINT ( 'NONE',  ( -5.711843387010018702, 0.9046671180729746187, 13.01999999999999424 ) ) ;
#4428=CARTESIAN_POINT ( 'NONE',  ( -5.711843387010018702, 0.9046671180729746187, 13.01999999999999424 ) ) ;
#4429=CARTESIAN_POINT ( 'NONE',  ( -4.900535883036028828, 2.496947748567499126, 7.559999999999998721 ) ) ;
#4441=CARTESIAN_POINT ( 'NONE',  ( -3.279728542977953687, 3.411736077305369541, 9.503948283277974696 ) ) ;
#4453=CARTESIAN_POINT ( 'NONE',  ( 0.6162731882459174804, 4.458484982038668498, 14.71605171672202239 ) ) ;
#4456=CARTESIAN_POINT ( 'NONE',  ( -5.446173322633801384, -0.7727076532861678615, 3.483948283277976898 ) ) ;
#4466=CARTESIAN_POINT ( 'NONE',  ( -4.009529358847660596, 2.042957248827953265, 10.35999999999999943 ) ) ;
#4470=CARTESIAN_POINT ( 'NONE',  ( 2.042957248827968808, -4.009529358847652603, 6.439999999999999503 ) ) ;
#4479=CARTESIAN_POINT ( 'NONE',  ( -0.9968613283357868893, 5.697241258616382531, 6.176051716722023244 ) ) ;
#4480=CARTESIAN_POINT ( 'NONE',  ( 5.711843387010018702, -0.9046671180729751738, 8.820000000000000284 ) ) ;
#4481=CARTESIAN_POINT ( 'NONE',  ( -0.9046671180729963790, 5.711843387010016926, 10.77999999999999936 ) ) ;
#4495=CARTESIAN_POINT ( 'NONE',  ( -3.244753828200538148, -3.119207202478392116, 8.803948283277977183 ) ) ;
#4507=CARTESIAN_POINT ( 'NONE',  ( 4.444597532678119300, 0.7039550926810472786, 0.2799999999999999711 ) ) ;
#4509=CARTESIAN_POINT ( 'NONE',  ( 4.458484982038663169, 0.6162731882459350219, 10.48394828327797512 ) ) ;
#4521=CARTESIAN_POINT ( 'NONE',  ( -4.673326407553653361, 0.7401821875142517992, 1.819999999999999396 ) ) ;
#4529=CARTESIAN_POINT ( 'NONE',  ( -0.7727076532861475444, -5.446173322633804048, 10.51605171672202133 ) ) ;
#4542=CARTESIAN_POINT ( 'NONE',  ( 5.446173322633801384, 0.7727076532861675284, 2.083948283277976543 ) ) ;
#4547=DIRECTION ( 'NONE',  ( 1.000000000000000000, 0.000000000000000000, 0.000000000000000000 ) ) ;
#4550=CARTESIAN_POINT ( 'NONE',  ( 3.889087296526005488, 3.889087296526018811, 13.99999999999999822 ) ) ;
#4551=CLOSED_SHELL ( 'NONE', ( #9403, #642, #4154, #4376 ) ) ;
#4556=CARTESIAN_POINT ( 'NONE',  ( 3.119207202478379681, 3.244753828200549695, 12.19605171672202282 ) ) ;
#4559=CARTESIAN_POINT ( 'NONE',  ( 2.417848759854264618, -4.940838830814695548, 11.04394828327797562 ) ) ;
#4569=MECHANICAL_DESIGN_GEOMETRIC_PRESENTATION_REPRESENTATION('',(#4235),#1187);
#4572=CARTESIAN_POINT ( 'NONE',  ( -3.345732310141667831, 3.345732310141653620, 4.900000000000000355 ) ) ;
#4583=CARTESIAN_POINT ( 'NONE',  ( -4.940838830814703542, 2.417848759854245078, 11.35605171672202296 ) ) ;
#4596=CARTESIAN_POINT ( 'NONE',  ( -5.697241258616385196, 0.9968613283357647958, 3.623948283277976135 ) ) ;
#4609=CARTESIAN_POINT ( 'NONE',  ( -4.009529358847660596, 2.042957248827953265, 4.759999999999999787 ) ) ;
#4612=CARTESIAN_POINT ( 'NONE',  ( 4.023224611898322145, -4.155232146225737111, 10.90394828327797327 ) ) ;
#4624=CARTESIAN_POINT ( 'NONE',  ( -4.215868657802586128, -2.148092372876348133, 7.139999999999997016 ) ) ;
#4632=CARTESIAN_POINT ( 'NONE',  ( -0.7727076532861475444, -5.446173322633804048, 13.31605171672202204 ) ) ;
#4634=CARTESIAN_POINT ( 'NONE',  ( 3.889087296526005488, 3.889087296526018811, 13.99999999999999822 ) ) ;
#4638=CARTESIAN_POINT ( 'NONE',  ( 0.9968613283357860011, -5.697241258616382531, 10.37605171672202253 ) ) ;
#4649=CARTESIAN_POINT ( 'NONE',  ( -0.9480714621563718358, -5.418398423912716311, 5.723948283277976223 ) ) ;
#4661=CARTESIAN_POINT ( 'NONE',  ( 4.215868657802586128, 2.148092372876346801, 8.539999999999999147 ) ) ;
#4664=CARTESIAN_POINT ( 'NONE',  ( 0.9480714621563713917, 5.418398423912717199, 12.72394828327797711 ) ) ;
#4668=SHAPE_DEFINITION_REPRESENTATION ( #10389, #7608 ) ;
#4679=CARTESIAN_POINT ( 'NONE',  ( 3.181980515339458471, 3.181980515339470461, 11.19999999999999751 ) ) ;
#4687=CARTESIAN_POINT ( 'NONE',  ( 5.726445515403654873, -0.8124729078101852187, 7.016051716722022213 ) ) ;
#4692=CARTESIAN_POINT ( 'NONE',  ( 2.542276634908080535, 5.195105386651229118, 12.05605171672202047 ) ) ;
#4693=ORIENTED_EDGE ( 'NONE', *, *, #6417, .F. ) ;
#4699=CARTESIAN_POINT ( 'NONE',  ( 4.860232935257354114, -2.576046737280751842, 2.363948283277975904 ) ) ;
#4711=CARTESIAN_POINT ( 'NONE',  ( 0.7039550926810297371, 4.444597532678122853, 5.319999999999999396 ) ) ;
#4715=CARTESIAN_POINT ( 'NONE',  ( 2.417848759854264618, -4.940838830814695548, 5.443948283277975975 ) ) ;
#4720=CARTESIAN_POINT ( 'NONE',  ( -0.8603895577212598011, -5.432285873273260179, 1.119999999999999885 ) ) ;
#4730=CARTESIAN_POINT ( 'NONE',  ( 3.181980515339458471, 3.181980515339470461, 8.400000000000000355 ) ) ;
#4749=CARTESIAN_POINT ( 'NONE',  ( 0.8323763977770604061, -4.658724279160015413, 1.976051716722022844 ) ) ;
#4763=CARTESIAN_POINT ( 'NONE',  ( -2.708615832122950096, -5.110351332421780413, 0.2639482832779765920 ) ) ;
#4773=CARTESIAN_POINT ( 'NONE',  ( -4.673326407553653361, 0.7401821875142517992, 4.620000000000000107 ) ) ;
#4774=ORIENTED_EDGE ( 'NONE', *, *, #5513, .F. ) ;
#4778=CARTESIAN_POINT ( 'NONE',  ( 5.697241258616385196, -0.9968613283357656840, 7.823948283277974980 ) ) ;
#4792=CARTESIAN_POINT ( 'NONE',  ( 4.215868657802586128, 2.148092372876346801, 11.33999999999999808 ) ) ;
#4804=CARTESIAN_POINT ( 'NONE',  ( -4.940838830814703542, 2.417848759854245078, 14.15605171672202012 ) ) ;
#4811=CARTESIAN_POINT ( 'NONE',  ( 3.889087296526005488, 3.889087296526018811, 8.400000000000000355 ) ) ;
#4814=CARTESIAN_POINT ( 'NONE',  ( -0.8603895577212598011, -5.432285873273260179, 1.119999999999999885 ) ) ;
#4826=CARTESIAN_POINT ( 'NONE',  ( 4.009529358847659708, -2.042957248827953709, 8.959999999999999076 ) ) ;
#4830=CARTESIAN_POINT ( 'NONE',  ( 0.9046671180729951578, -5.711843387010016926, 3.779999999999998472 ) ) ;
#4843=CARTESIAN_POINT ( 'NONE',  ( -4.009529358847660596, 2.042957248827953265, 10.35999999999999943 ) ) ;
#4851=CARTESIAN_POINT ( 'NONE',  ( -4.673326407553653361, 0.7401821875142517992, 1.819999999999999618 ) ) ;
#4854=CARTESIAN_POINT ( 'NONE',  ( 0.7727076532861471003, 5.446173322633805824, 11.91605171672202346 ) ) ;
#4862=CARTESIAN_POINT ( 'NONE',  ( -5.152728359536494551, -2.625446233515535077, 7.139999999999997016 ) ) ;
#4864=CARTESIAN_POINT ( 'NONE',  ( 2.496947748567516889, -4.900535883036019946, 0.8399999999999999689 ) ) ;
#4877=CARTESIAN_POINT ( 'NONE',  ( 4.658724279160018966, -0.8323763977770426425, 5.023948283277976046 ) ) ;
#4880=CARTESIAN_POINT ( 'NONE',  ( 2.625446233515515537, 5.152728359536502545, 8.259999999999999787 ) ) ;
#4889=CARTESIAN_POINT ( 'NONE',  ( 0.7727076532861471003, 5.446173322633805824, 14.71605171672202239 ) ) ;
#4892=CARTESIAN_POINT ( 'NONE',  ( -0.7916369971161423269, -4.430710083317576320, 2.923948283277976401 ) ) ;
#4903=CARTESIAN_POINT ( 'NONE',  ( 2.042957248827968808, -4.009529358847652603, 0.8399999999999999689 ) ) ;
#4907=CARTESIAN_POINT ( 'NONE',  ( -4.049832306626335310, 1.963858260114700327, 8.556051716722022249 ) ) ;
#4916=CARTESIAN_POINT ( 'NONE',  ( 2.496947748567516889, -4.900535883036019946, 0.8399999999999999689 ) ) ;
#4917=DIRECTION ( 'NONE',  ( 0.7071067811865467956, 0.7071067811865484609, 0.000000000000000000 ) ) ;
#4918=CARTESIAN_POINT ( 'NONE',  ( -5.195105386651219348, -2.542276634908102295, 11.74394828327797846 ) ) ;
#4933=CARTESIAN_POINT ( 'NONE',  ( -4.458484982038663169, -0.6162731882459353550, 3.483948283277976898 ) ) ;
#4938=CARTESIAN_POINT ( 'NONE',  ( 5.432285873273257515, 0.8603895577212793411, 8.679999999999997939 ) ) ;
#4940=CARTESIAN_POINT ( 'NONE',  ( 3.889087296526005488, 3.889087296526018811, 8.400000000000000355 ) ) ;
#4945=CARTESIAN_POINT ( 'NONE',  ( 3.119207202478379681, 3.244753828200549695, 6.596051716722022285 ) ) ;
#4948=CARTESIAN_POINT ( 'NONE',  ( 1.963858260114715870, -4.049832306626327316, 8.243948283277976685 ) ) ;
#4959=CARTESIAN_POINT ( 'NONE',  ( 0.6162731882459174804, 4.458484982038668498, 9.116051716722020970 ) ) ;
#4968=CARTESIAN_POINT ( 'NONE',  ( 5.432285873273257515, 0.8603895577212793411, 0.2799999999999999156 ) ) ;
#4969=CARTESIAN_POINT ( 'NONE',  ( 5.711843387010018702, -0.9046671180729751738, 3.219999999999999751 ) ) ;
#4970=CARTESIAN_POINT ( 'NONE',  ( -4.860232935257354114, 2.576046737280751842, 9.363948283277975904 ) ) ;
#4983=CARTESIAN_POINT ( 'NONE',  ( -4.658724279160018078, 0.8323763977770419764, 0.8239482832779764232 ) ) ;
#4986=CARTESIAN_POINT ( 'NONE',  ( -3.889087296526005044, -3.889087296526019255, 1.399999999999999689 ) ) ;
#4990=CARTESIAN_POINT ( 'NONE',  ( 2.496947748567516889, -4.900535883036019946, 12.03999999999999915 ) ) ;
#4998=CARTESIAN_POINT ( 'NONE',  ( 4.049832306626335310, -1.963858260114701215, 4.356051716722023848 ) ) ;
#5001=CARTESIAN_POINT ( 'NONE',  ( -2.231261971483764484, -4.173491630687871101, 8.663948283277974838 ) ) ;
#5005=CARTESIAN_POINT ( 'NONE',  ( 3.826313983664925811, 3.951860609387098044, 6.596051716722022285 ) ) ;
#5014=CARTESIAN_POINT ( 'NONE',  ( 3.119207202478379681, 3.244753828200549695, 12.19605171672202282 ) ) ;
#5023=CARTESIAN_POINT ( 'NONE',  ( -2.542276634908081423, -5.195105386651227342, 2.256051716722022871 ) ) ;
#5024=CARTESIAN_POINT ( 'NONE',  ( -0.8603895577212598011, -5.432285873273260179, 1.119999999999999885 ) ) ;
#5025=CARTESIAN_POINT ( 'NONE',  ( -0.8124729078102072011, 5.726445515403652209, 12.58394828327797477 ) ) ;
#5035=CARTESIAN_POINT ( 'NONE',  ( 3.969226411068985882, -2.122056237541205981, 2.363948283277975904 ) ) ;
#5038=CARTESIAN_POINT ( 'NONE',  ( -5.711843387010018702, 0.9046671180729746187, 4.620000000000000107 ) ) ;
#5040=CARTESIAN_POINT ( 'NONE',  ( 5.152728359536493663, 2.625446233515533745, 8.539999999999999147 ) ) ;
#5044=CARTESIAN_POINT ( 'NONE',  ( 4.173491630687861331, 2.231261971483781359, 3.936051716722023031 ) ) ;
#5047=CARTESIAN_POINT ( 'NONE',  ( 0.6479879772514793856, -4.687928535947285091, 2.783948283277976277 ) ) ;
#5050=CARTESIAN_POINT ( 'NONE',  ( -4.155232146225753098, 4.023224611898306158, 5.896051716722023883 ) ) ;
#5054=CARTESIAN_POINT ( 'NONE',  ( 0.7401821875142697849, -4.673326407553650697, 0.9799999999999997602 ) ) ;
#5060=CARTESIAN_POINT ( 'NONE',  ( 4.430710083317573655, 0.7916369971161595354, 12.47605171672202218 ) ) ;
#5068=CARTESIAN_POINT ( 'NONE',  ( 2.625446233515515537, 5.152728359536502545, 11.05999999999999872 ) ) ;
#5069=CARTESIAN_POINT ( 'NONE',  ( -0.9046671180729963790, 5.711843387010016926, 7.979999999999999538 ) ) ;
#5070=CARTESIAN_POINT ( 'NONE',  ( 2.496947748567516889, -4.900535883036019946, 12.03999999999999915 ) ) ;
#5084=CARTESIAN_POINT ( 'NONE',  ( 0.7401821875142697849, -4.673326407553650697, 12.17999999999999439 ) ) ;
#5088=CARTESIAN_POINT ( 'NONE',  ( -5.711843387010018702, 0.9046671180729746187, 10.21999999999999709 ) ) ;
#5092=CARTESIAN_POINT ( 'NONE',  ( 4.089228379062037178, -4.089228379062022967, 6.299999999999998934 ) ) ;
#5098=CARTESIAN_POINT ( 'NONE',  ( -4.173491630687863108, -2.231261971483782691, 5.336051716722022498 ) ) ;
#5101=CARTESIAN_POINT ( 'NONE',  ( -0.6479879772514802738, 4.687928535947285091, 1.383948283277976365 ) ) ;
#5105=CARTESIAN_POINT ( 'NONE',  ( 2.576046737280769605, -4.860232935257343456, 1.836051716722023386 ) ) ;
#5112=CARTESIAN_POINT ( 'NONE',  ( -4.049832306626335310, 1.963858260114700327, 5.756051716722022427 ) ) ;
#5120=CARTESIAN_POINT ( 'NONE',  ( 5.110351332421769754, 2.708615832122969191, 3.936051716722023031 ) ) ;
#5121=CARTESIAN_POINT ( 'NONE',  ( 5.711843387010018702, -0.9046671180729751738, 6.019999999999999574 ) ) ;
#5122=CARTESIAN_POINT ( 'NONE',  ( 4.089228379062037178, -4.089228379062022967, 6.299999999999999822 ) ) ;
#5133=DIRECTION ( 'NONE',  ( -0.7043149233066458015, 0.7043149233066440251, -0.08877487040322762368 ) ) ;
#5137=CARTESIAN_POINT ( 'NONE',  ( 4.658724279160018966, -0.8323763977770426425, 7.823948283277974980 ) ) ;
#5138=VERTEX_POINT ( 'NONE', #10195 ) ;
#5140=CARTESIAN_POINT ( 'NONE',  ( 5.711843387010018702, -0.9046671180729751738, 11.61999999999999922 ) ) ;
#5144=CARTESIAN_POINT ( 'NONE',  ( -5.432285873273256627, -0.8603895577212797852, 7.279999999999999361 ) ) ;
#5148=CARTESIAN_POINT ( 'NONE',  ( -4.673326407553653361, 0.7401821875142517992, 1.819999999999999396 ) ) ;
#5150=CARTESIAN_POINT ( 'NONE',  ( -0.9480714621563718358, -5.418398423912716311, 2.923948283277976401 ) ) ;
#5154=CARTESIAN_POINT ( 'NONE',  ( 0.9968613283357860011, -5.697241258616382531, 1.976051716722022844 ) ) ;
#5161=CARTESIAN_POINT ( 'NONE',  ( -4.444597532678119300, -0.7039550926810477227, 10.07999999999999829 ) ) ;
#5163=CARTESIAN_POINT ( 'NONE',  ( -2.064922774268895811, -4.258245684917318918, 13.45605171672202260 ) ) ;
#5172=CARTESIAN_POINT ( 'NONE',  ( -0.8603895577212598011, -5.432285873273260179, 12.31999999999999851 ) ) ;
#5173=CARTESIAN_POINT ( 'NONE',  ( 0.8603895577212593571, 5.432285873273261068, 2.519999999999999574 ) ) ;
#5174=CARTESIAN_POINT ( 'NONE',  ( -4.900535883036028828, 2.496947748567499126, 10.35999999999999943 ) ) ;
#5188=CARTESIAN_POINT ( 'NONE',  ( 5.446173322633801384, 0.7727076532861675284, -0.7160517167220232793 ) ) ;
#5199=CARTESIAN_POINT ( 'NONE',  ( -2.122056237541221968, 3.969226411068977889, 8.836051716722023386 ) ) ;
#5202=CARTESIAN_POINT ( 'NONE',  ( 5.697241258616385196, -0.9968613283357656840, 2.223948283277975779 ) ) ;
#5205=CARTESIAN_POINT ( 'NONE',  ( -4.940838830814703542, 2.417848759854245078, 2.956051716722023492 ) ) ;
#5209=CARTESIAN_POINT ( 'NONE',  ( -3.345732310141667831, 3.345732310141653620, 10.50000000000000000 ) ) ;
#5211=CARTESIAN_POINT ( 'NONE',  ( 4.215868657802586128, 2.148092372876346801, 5.739999999999997549 ) ) ;
#5221=CARTESIAN_POINT ( 'NONE',  ( 4.900535883036028828, -2.496947748567499126, 11.75999999999999979 ) ) ;
#5224=CARTESIAN_POINT ( 'NONE',  ( -2.625446233515515981, -5.152728359536500768, 9.659999999999994813 ) ) ;
#5225=CARTESIAN_POINT ( 'NONE',  ( 5.711843387010018702, -0.9046671180729751738, 6.019999999999999574 ) ) ;
#5241=CARTESIAN_POINT ( 'NONE',  ( 3.969226411068985882, -2.122056237541205981, 7.963948283277976437 ) ) ;
#5256=CARTESIAN_POINT ( 'NONE',  ( -2.064922774268895811, -4.258245684917318918, 13.45605171672202260 ) ) ;
#5260=CARTESIAN_POINT ( 'NONE',  ( -4.658724279160018078, 0.8323763977770419764, 12.02394828327797427 ) ) ;
#5271=CARTESIAN_POINT ( 'NONE',  ( 2.042957248827968808, -4.009529358847652603, 9.240000000000000213 ) ) ;
#5272=CARTESIAN_POINT ( 'NONE',  ( 4.673326407553653361, -0.7401821875142523544, 3.219999999999999751 ) ) ;
#5274=ORIENTED_EDGE ( 'NONE', *, *, #1169, .T. ) ;
#5281=CARTESIAN_POINT ( 'NONE',  ( 0.9968613283357860011, -5.697241258616382531, 7.576051716722023599 ) ) ;
#5282=CARTESIAN_POINT ( 'NONE',  ( -5.432285873273256627, -0.8603895577212797852, 10.07999999999999829 ) ) ;
#5283=CARTESIAN_POINT ( 'NONE',  ( 2.625446233515515537, 5.152728359536502545, 5.459999999999997300 ) ) ;
#5294=CARTESIAN_POINT ( 'NONE',  ( 4.258245684917310037, 2.064922774268912686, 7.543948283277975619 ) ) ;
#5306=CARTESIAN_POINT ( 'NONE',  ( 2.042957248827968808, -4.009529358847652603, 0.8399999999999999689 ) ) ;
#5308=CARTESIAN_POINT ( 'NONE',  ( -4.258245684917310925, -2.064922774268914019, 11.74394828327797846 ) ) ;
#5319=CARTESIAN_POINT ( 'NONE',  ( -3.181980515339458027, -3.181980515339470905, 1.399999999999999689 ) ) ;
#5330=CARTESIAN_POINT ( 'NONE',  ( 2.542276634908080535, 5.195105386651229118, 12.05605171672202047 ) ) ;
#5344=CARTESIAN_POINT ( 'NONE',  ( -4.860232935257354114, 2.576046737280751842, 6.563948283277975193 ) ) ;
#5354=CARTESIAN_POINT ( 'NONE',  ( 3.119207202478379681, 3.244753828200549695, 14.99605171672202175 ) ) ;
#5355=( BOUNDED_CURVE ( )  B_SPLINE_CURVE ( 2, ( #8151, #6438, #7450, #193, #91, #4111, #4903, #5054, #9698, #2424, #3266, #9851, #3421, #4851, #3317, #5641, #4011, #1731, #7239, #8096, #6644, #6543, #9794, #933, #825, #4056, #7293, #40, #6489, #2522, #9746, #5741, #2577, #2476, #5792, #9046, #5690, #1675, #3365, #8991, #7397, #139, #4360, #3472, #4309, #7601, #348, #6046, #5945, #298, #1137, #9253, #1086, #2041, #6698, #1989, #2093, #8509, #3574, #9952, #7556, #2832, #6799, #10056, #3623, #5995, #5271, #2781, #10004, #450, #3521, #9144, #5161, #6742, #4466, #5209, #4258, #8456, #1188, #7657, #7503, #4415, #8410, #245, #2730, #9198, #1937, #2677, #396, #6852, #10107, #9300, #1241, #7715, #3675, #6903, #10157, #2882, #6109, #5891, #9358 ),
 .UNSPECIFIED., .F., .T. ) 
 B_SPLINE_CURVE_WITH_KNOTS ( ( 3, 2, 2, 2, 2, 2, 2, 2, 2, 2, 2, 2, 2, 2, 2, 2, 2, 2, 2, 2, 2, 2, 2, 2, 2, 2, 2, 2, 2, 2, 2, 2, 2, 2, 2, 2, 2, 2, 2, 2, 2, 2, 2, 2, 2, 2, 2, 2, 2, 2, 3 ),
 ( 0.000000000000000000, 0.02000000000000000042, 0.04000000000000000083, 0.05999999999999999778, 0.08000000000000000167, 0.1000000000000000056, 0.1199999999999999956, 0.1400000000000000133, 0.1600000000000000033, 0.1799999999999999933, 0.2000000000000000111, 0.2200000000000000011, 0.2399999999999999911, 0.2600000000000000089, 0.2800000000000000266, 0.2999999999999999889, 0.3200000000000000067, 0.3400000000000000244, 0.3599999999999999867, 0.3800000000000000044, 0.4000000000000000222, 0.4199999999999999845, 0.4400000000000000022, 0.4600000000000000200, 0.4799999999999999822, 0.5000000000000000000, 0.5200000000000000178, 0.5400000000000000355, 0.5600000000000000533, 0.5799999999999999600, 0.5999999999999999778, 0.6199999999999999956, 0.6400000000000000133, 0.6600000000000000311, 0.6800000000000000488, 0.6999999999999999556, 0.7199999999999999734, 0.7399999999999999911, 0.7600000000000000089, 0.7800000000000000266, 0.8000000000000000444, 0.8199999999999999512, 0.8399999999999999689, 0.8599999999999999867, 0.8800000000000000044, 0.9000000000000000222, 0.9200000000000000400, 0.9399999999999999467, 0.9599999999999999645, 0.9799999999999999822, 1.000000000000000000 ),
 .UNSPECIFIED. ) 
 CURVE ( )  GEOMETRIC_REPRESENTATION_ITEM ( )  RATIONAL_B_SPLINE_CURVE ( ( 1.000000000000000000, 0.9510565162951535312, 1.000000000000000000, 0.9510565162951535312, 1.000000000000000000, 0.9510565162951535312, 1.000000000000000000, 0.9510565162951535312, 1.000000000000000000, 0.9510565162951535312, 1.000000000000000000, 0.9510565162951535312, 1.000000000000000000, 0.9510565162951535312, 1.000000000000000000, 0.9510565162951535312, 1.000000000000000000, 0.9510565162951535312, 1.000000000000000000, 0.9510565162951535312, 1.000000000000000000, 0.9510565162951535312, 1.000000000000000000, 0.9510565162951535312, 1.000000000000000000, 0.9510565162951535312, 1.000000000000000000, 0.9510565162951535312, 1.000000000000000000, 0.9510565162951535312, 1.000000000000000000, 0.9510565162951535312, 1.000000000000000000, 0.9510565162951535312, 1.000000000000000000, 0.9510565162951535312, 1.000000000000000000, 0.9510565162951535312, 1.000000000000000000, 0.9510565162951535312, 1.000000000000000000, 0.9510565162951535312, 1.000000000000000000, 0.9510565162951535312, 1.000000000000000000, 0.9510565162951535312, 1.000000000000000000, 0.9510565162951535312, 1.000000000000000000, 0.9510565162951535312, 1.000000000000000000, 0.9510565162951535312, 1.000000000000000000, 0.9510565162951535312, 1.000000000000000000, 0.9510565162951535312, 1.000000000000000000, 0.9510565162951535312, 1.000000000000000000, 0.9510565162951535312, 1.000000000000000000, 0.9510565162951535312, 1.000000000000000000, 0.9510565162951535312, 1.000000000000000000, 0.9510565162951535312, 1.000000000000000000, 0.9510565162951535312, 1.000000000000000000, 0.9510565162951535312, 1.000000000000000000, 0.9510565162951535312, 1.000000000000000000, 0.9510565162951535312, 1.000000000000000000, 0.9510565162951535312, 1.000000000000000000, 0.9510565162951535312, 1.000000000000000000, 0.9510565162951535312, 1.000000000000000000, 0.9510565162951535312, 1.000000000000000000, 0.9510565162951535312, 1.000000000000000000, 0.9510565162951535312, 1.000000000000000000, 0.9510565162951535312, 1.000000000000000000, 0.9510565162951535312, 1.000000000000000000, 0.9510565162951535312, 1.000000000000000000, 0.9510565162951535312, 1.000000000000000000, 0.9510565162951535312, 1.000000000000000000, 0.9510565162951535312, 1.000000000000000000, 0.9510565162951535312, 1.000000000000000000 ) ) 
 REPRESENTATION_ITEM ( '' )  );
#5358=CARTESIAN_POINT ( 'NONE',  ( -3.969226411068985882, 2.122056237541205537, 12.16394828327797661 ) ) ;
#5369=CARTESIAN_POINT ( 'NONE',  ( -0.7401821875142701179, 4.673326407553649808, 5.179999999999999716 ) ) ;
#5377=CARTESIAN_POINT ( 'NONE',  ( 4.155232146225751322, -4.023224611898307934, 10.09605171672202140 ) ) ;
#5383=SURFACE_STYLE_USAGE ( .BOTH. , #2214 ) ;
#5388=VERTEX_POINT ( 'NONE', #3296 ) ;
#5392=CARTESIAN_POINT ( 'NONE',  ( -0.9480714621563718358, -5.418398423912716311, 8.523948283277976046 ) ) ;
#5405=CARTESIAN_POINT ( 'NONE',  ( -2.042957248827969252, 4.009529358847651714, 5.039999999999999147 ) ) ;
#5408=CARTESIAN_POINT ( 'NONE',  ( -4.023224611898323033, 4.155232146225737111, 12.30394828327797718 ) ) ;
#5413=( BOUNDED_SURFACE ( )  B_SPLINE_SURFACE ( 3, 2, ( 
 ( #9544, #1690, #4968, #2435, #7196, #3278, #4916, #3221, #7249, #3300, #4120, #6500, #8213, #2590, #5700, #9758, #6607, #9864, #6554, #10453, #2487, #8164, #6451, #9708, #5654, #7359, #8946, #947, #5805, #894, #102, #9057, #1795, #9807, #3329, #2536, #5755, #9004, #1741, #7408, #149, #8898, #4173, #3380, #8003, #1640, #4020, #735, #2378, #3967, #3170, #4862, #6394, #9651, #8107, #839, #5605, #4070, #8848, #1589, #4811, #7307, #49, #8059, #790, #4271, #10019, #9262, #3586, #6009, #5857, #8368, #7465, #3636, #5955, #6866, #9109, #2002, #10120, #5068, #9313, #1097, #308, #2640, #5221, #8471, #1845, #1949, #5172, #9210, #6811, #1203, #8421, #4427, #2842, #208, #4222, #5907, #1147, #4370, #6058 ),
 ( #2791, #2688, #7516, #4321, #7617, #8320, #7672, #3432, #360, #5023, #410, #8267, #992, #3484, #10067, #6655, #9912, #1050, #257, #6707, #9965, #5120, #9160, #1900, #7565, #3531, #6757, #2744, #2055, #2208, #6328, #2105, #6118, #7773, #10383, #9475, #2156, #4479, #506, #6219, #9533, #6968, #1464, #4687, #3739, #7019, #8722, #5281, #1303, #8573, #7071, #6913, #3106, #2260, #10222, #1254, #7727, #2952, #6171, #460, #9427, #3687, #6277, #5483, #1355, #5377, #8616, #10169, #4529, #10275, #7931, #615, #3055, #2897, #4583, #9370, #663, #3004, #3897, #5330, #7127, #8522, #7829, #561, #3789, #5435, #8673, #1407, #4632, #7879, #3843, #10320, #178, #8292, #3460, #9888, #9942, #1075, #4889, #8777, #128 ),
 ( #8190, #235, #76, #1821, #3303, #2617, #2666, #919, #3511, #5834, #9087, #6530, #5881, #8978, #8138, #4148, #9783, #6683, #4248, #8244, #1769, #5044, #7434, #9130, #4998, #7385, #1873, #2512, #5726, #6580, #1721, #5098, #5781, #5536, #3412, #2567, #1019, #1518, #4297, #9032, #4945, #3353, #873, #971, #9837, #7493, #4197, #7542, #9586, #7333, #8346, #4100, #6635, #286, #2313, #2026, #5199, #6727, #8444, #8596, #3664, #1327, #2133, #7589, #3611, #1979, #8396, #6838, #1281, #9187, #7648, #1174, #385, #10199, #9990, #6892, #539, #6789, #332, #4402, #4556, #10145, #10095, #1925, #2822, #438, #3712, #6035, #5935, #5256, #2868, #9287, #5982, #9240, #6092, #8497, #6944, #7805, #4453, #1228, #5354 ),
 ( #7701, #9346, #4507, #6146, #9396, #2080, #5306, #2927, #2716, #8547, #2769, #7752, #1127, #5148, #4348, #486, #3561, #10046, #2238, #8698, #9452, #638, #6199, #8018, #751, #3082, #3868, #7907, #2181, #3027, #8752, #3984, #2340, #4773, #4609, #7100, #5405, #2397, #4711, #5617, #7851, #7215, #8861, #3818, #8073, #10358, #9561, #1385, #10468, #3185, #587, #699, #3928, #7962, #5562, #6407, #7155, #9667, #1603, #8649, #2980, #4661, #10412, #3133, #4826, #3764, #6995, #5459, #6302, #1551, #1435, #6248, #2288, #6361, #7047, #10247, #10299, #9613, #9508, #5512, #1491, #8807, #9773, #3396, #3240, #6625, #7421, #5084, #4237, #9018, #4134, #164, #7261, #5871, #7373, #4087, #8121, #6463, #3341, #8961, #5822 ),
 ( #64, #3290, #9876, #9820, #8281, #9121, #1756, #2552, #9929, #2656, #2606, #5769, #9075, #4983, #6569, #1810, #223, #3448, #2501, #8230, #7483, #804, #6516, #7321, #5035, #5665, #1861, #1007, #1704, #9, #9720, #5714, #4933, #2451, #8176, #8914, #6671, #4032, #117, #908, #961, #1652, #4187, #4877, #855, #6881, #9334, #9177, #1161, #273, #6927, #9276, #10187, #1915, #2070, #2915, #8383, #2119, #4388, #3600, #5921, #5294, #8536, #5137, #5241, #8486, #2015, #10135, #1268, #1218, #4495, #6132, #3500, #7528, #9226, #4441, #7689, #9384, #8337, #7740, #10036, #7635, #6078, #5972, #321, #375, #425, #1113, #475, #6717, #3654, #1064, #3699, #4287, #9978, #6773, #2856, #2702, #4338, #7578, #3548 ),
 ( #2757, #1966, #5188, #8435, #6826, #10083, #2810, #6025, #575, #4763, #8793, #3803, #1477, #8005, #738, #3017, #2966, #6234, #6290, #3969, #8740, #2328, #4542, #10236, #4699, #9546, #8686, #7086, #7198, #3858, #7945, #3119, #10455, #4596, #7788, #3172, #682, #5550, #7036, #3915, #5446, #6397, #1422, #9600, #2274, #7839, #524, #10400, #4649, #8586, #6346, #10287, #7141, #6187, #5344, #1371, #7895, #3752, #629, #1535, #9493, #9653, #1317, #9441, #6983, #2169, #2226, #10341, #5392, #8633, #3071, #5498, #3382, #3223, #4970, #6453, #2538, #2593, #4072, #6657, #5757, #9006, #9710, #9060, #1642, #792, #841, #2437, #9865, #7410, #896, #4918, #8216, #104, #6610, #8166, #7309, #5025, #5656, #8901, #9760 ),
 ( #3331, #5702, #1743, #8850, #7468, #8948, #4864, #8109, #4814, #4122, #51, #152, #3280, #210, #2380, #1786, #949, #7251, #7362, #4022, #5807, #6557, #6503, #5607, #2490, #4225, #9809, #3434, #8269, #1692, #4175, #1797, #994, #1591, #8061, #1256, #8423, #9264, #7674, #5283, #9164, #9111, #9316, #5225, #6868, #5122, #2004, #10022, #7730, #2746, #3640, #363, #1903, #1847, #4429, #5958, #2643, #412, #8370, #1206, #7518, #9915, #5909, #9212, #8324, #1952, #8473, #1099, #10122, #2844, #4273, #6061, #2058, #4323, #5174, #3689, #6709, #4481, #7567, #8524, #261, #462, #3487, #10070, #5859, #310, #5070, #2795, #6011, #9967, #1052, #3534, #2690, #6759, #1149, #4373, #7619, #3588, #6813, #2261, #4634 ) ),
 .UNSPECIFIED., .T., .F., .T. ) 
 B_SPLINE_SURFACE_WITH_KNOTS ( ( 4, 3, 4 ),
 ( 3, 2, 2, 2, 2, 2, 2, 2, 2, 2, 2, 2, 2, 2, 2, 2, 2, 2, 2, 2, 2, 2, 2, 2, 2, 2, 2, 2, 2, 2, 2, 2, 2, 2, 2, 2, 2, 2, 2, 2, 2, 2, 2, 2, 2, 2, 2, 2, 2, 2, 3 ),
 ( 0.000000000000000000, 0.5000000000000000000, 1.000000000000000000 ),
 ( 0.000000000000000000, 0.02000000000000000042, 0.04000000000000000083, 0.05999999999999999778, 0.08000000000000000167, 0.1000000000000000056, 0.1199999999999999956, 0.1400000000000000133, 0.1600000000000000033, 0.1799999999999999933, 0.2000000000000000111, 0.2200000000000000011, 0.2399999999999999911, 0.2600000000000000089, 0.2800000000000000266, 0.2999999999999999889, 0.3200000000000000067, 0.3400000000000000244, 0.3599999999999999867, 0.3800000000000000044, 0.4000000000000000222, 0.4199999999999999845, 0.4400000000000000022, 0.4600000000000000200, 0.4799999999999999822, 0.5000000000000000000, 0.5200000000000000178, 0.5400000000000000355, 0.5600000000000000533, 0.5799999999999999600, 0.5999999999999999778, 0.6199999999999999956, 0.6400000000000000133, 0.6600000000000000311, 0.6800000000000000488, 0.6999999999999999556, 0.7199999999999999734, 0.7399999999999999911, 0.7600000000000000089, 0.7800000000000000266, 0.8000000000000000444, 0.8199999999999999512, 0.8399999999999999689, 0.8599999999999999867, 0.8800000000000000044, 0.9000000000000000222, 0.9200000000000000400, 0.9399999999999999467, 0.9599999999999999645, 0.9799999999999999822, 1.000000000000000000 ),
 .UNSPECIFIED. ) 
 GEOMETRIC_REPRESENTATION_ITEM ( )  RATIONAL_B_SPLINE_SURFACE ( (
 ( 1.000000000000000000, 0.9510565162951535312, 1.000000000000000000, 0.9510565162951535312, 1.000000000000000000, 0.9510565162951535312, 1.000000000000000000, 0.9510565162951535312, 1.000000000000000000, 0.9510565162951535312, 1.000000000000000000, 0.9510565162951535312, 1.000000000000000000, 0.9510565162951535312, 1.000000000000000000, 0.9510565162951535312, 1.000000000000000000, 0.9510565162951535312, 1.000000000000000000, 0.9510565162951535312, 1.000000000000000000, 0.9510565162951535312, 1.000000000000000000, 0.9510565162951535312, 1.000000000000000000, 0.9510565162951535312, 1.000000000000000000, 0.9510565162951535312, 1.000000000000000000, 0.9510565162951535312, 1.000000000000000000, 0.9510565162951535312, 1.000000000000000000, 0.9510565162951535312, 1.000000000000000000, 0.9510565162951535312, 1.000000000000000000, 0.9510565162951535312, 1.000000000000000000, 0.9510565162951535312, 1.000000000000000000, 0.9510565162951535312, 1.000000000000000000, 0.9510565162951535312, 1.000000000000000000, 0.9510565162951535312, 1.000000000000000000, 0.9510565162951535312, 1.000000000000000000, 0.9510565162951535312, 1.000000000000000000, 0.9510565162951535312, 1.000000000000000000, 0.9510565162951535312, 1.000000000000000000, 0.9510565162951535312, 1.000000000000000000, 0.9510565162951535312, 1.000000000000000000, 0.9510565162951535312, 1.000000000000000000, 0.9510565162951535312, 1.000000000000000000, 0.9510565162951535312, 1.000000000000000000, 0.9510565162951535312, 1.000000000000000000, 0.9510565162951535312, 1.000000000000000000, 0.9510565162951535312, 1.000000000000000000, 0.9510565162951535312, 1.000000000000000000, 0.9510565162951535312, 1.000000000000000000, 0.9510565162951535312, 1.000000000000000000, 0.9510565162951535312, 1.000000000000000000, 0.9510565162951535312, 1.000000000000000000, 0.9510565162951535312, 1.000000000000000000, 0.9510565162951535312, 1.000000000000000000, 0.9510565162951535312, 1.000000000000000000, 0.9510565162951535312, 1.000000000000000000, 0.9510565162951535312, 1.000000000000000000, 0.9510565162951535312, 1.000000000000000000, 0.9510565162951535312, 1.000000000000000000, 0.9510565162951535312, 1.000000000000000000, 0.9510565162951535312, 1.000000000000000000, 0.9510565162951535312, 1.000000000000000000),
 ( 0.3333333333333333703, 0.3170188387650512141, 0.3333333333333333703, 0.3170188387650512141, 0.3333333333333333703, 0.3170188387650512141, 0.3333333333333333703, 0.3170188387650512141, 0.3333333333333333703, 0.3170188387650512141, 0.3333333333333333703, 0.3170188387650512141, 0.3333333333333333703, 0.3170188387650512141, 0.3333333333333333703, 0.3170188387650512141, 0.3333333333333333703, 0.3170188387650512141, 0.3333333333333333703, 0.3170188387650512141, 0.3333333333333333703, 0.3170188387650512141, 0.3333333333333333703, 0.3170188387650512141, 0.3333333333333333703, 0.3170188387650512141, 0.3333333333333333703, 0.3170188387650512141, 0.3333333333333333703, 0.3170188387650512141, 0.3333333333333333703, 0.3170188387650512141, 0.3333333333333333703, 0.3170188387650512141, 0.3333333333333333703, 0.3170188387650512141, 0.3333333333333333703, 0.3170188387650512141, 0.3333333333333333703, 0.3170188387650512141, 0.3333333333333333703, 0.3170188387650512141, 0.3333333333333333703, 0.3170188387650512141, 0.3333333333333333703, 0.3170188387650512141, 0.3333333333333333703, 0.3170188387650512141, 0.3333333333333333703, 0.3170188387650512141, 0.3333333333333333703, 0.3170188387650512141, 0.3333333333333333703, 0.3170188387650512141, 0.3333333333333333703, 0.3170188387650512141, 0.3333333333333333703, 0.3170188387650512141, 0.3333333333333333703, 0.3170188387650512141, 0.3333333333333333703, 0.3170188387650512141, 0.3333333333333333703, 0.3170188387650512141, 0.3333333333333333703, 0.3170188387650512141, 0.3333333333333333703, 0.3170188387650512141, 0.3333333333333333703, 0.3170188387650512141, 0.3333333333333333703, 0.3170188387650512141, 0.3333333333333333703, 0.3170188387650512141, 0.3333333333333333703, 0.3170188387650512141, 0.3333333333333333703, 0.3170188387650512141, 0.3333333333333333703, 0.3170188387650512141, 0.3333333333333333703, 0.3170188387650512141, 0.3333333333333333703, 0.3170188387650512141, 0.3333333333333333703, 0.3170188387650512141, 0.3333333333333333703, 0.3170188387650512141, 0.3333333333333333703, 0.3170188387650512141, 0.3333333333333333703, 0.3170188387650512141, 0.3333333333333333703, 0.3170188387650512141, 0.3333333333333333703, 0.3170188387650512141, 0.3333333333333333703, 0.3170188387650512141, 0.3333333333333333703, 0.3170188387650512141, 0.3333333333333333703),
 ( 0.3333333333333333703, 0.3170188387650512141, 0.3333333333333333703, 0.3170188387650512141, 0.3333333333333333703, 0.3170188387650512141, 0.3333333333333333703, 0.3170188387650512141, 0.3333333333333333703, 0.3170188387650512141, 0.3333333333333333703, 0.3170188387650512141, 0.3333333333333333703, 0.3170188387650512141, 0.3333333333333333703, 0.3170188387650512141, 0.3333333333333333703, 0.3170188387650512141, 0.3333333333333333703, 0.3170188387650512141, 0.3333333333333333703, 0.3170188387650512141, 0.3333333333333333703, 0.3170188387650512141, 0.3333333333333333703, 0.3170188387650512141, 0.3333333333333333703, 0.3170188387650512141, 0.3333333333333333703, 0.3170188387650512141, 0.3333333333333333703, 0.3170188387650512141, 0.3333333333333333703, 0.3170188387650512141, 0.3333333333333333703, 0.3170188387650512141, 0.3333333333333333703, 0.3170188387650512141, 0.3333333333333333703, 0.3170188387650512141, 0.3333333333333333703, 0.3170188387650512141, 0.3333333333333333703, 0.3170188387650512141, 0.3333333333333333703, 0.3170188387650512141, 0.3333333333333333703, 0.3170188387650512141, 0.3333333333333333703, 0.3170188387650512141, 0.3333333333333333703, 0.3170188387650512141, 0.3333333333333333703, 0.3170188387650512141, 0.3333333333333333703, 0.3170188387650512141, 0.3333333333333333703, 0.3170188387650512141, 0.3333333333333333703, 0.3170188387650512141, 0.3333333333333333703, 0.3170188387650512141, 0.3333333333333333703, 0.3170188387650512141, 0.3333333333333333703, 0.3170188387650512141, 0.3333333333333333703, 0.3170188387650512141, 0.3333333333333333703, 0.3170188387650512141, 0.3333333333333333703, 0.3170188387650512141, 0.3333333333333333703, 0.3170188387650512141, 0.3333333333333333703, 0.3170188387650512141, 0.3333333333333333703, 0.3170188387650512141, 0.3333333333333333703, 0.3170188387650512141, 0.3333333333333333703, 0.3170188387650512141, 0.3333333333333333703, 0.3170188387650512141, 0.3333333333333333703, 0.3170188387650512141, 0.3333333333333333703, 0.3170188387650512141, 0.3333333333333333703, 0.3170188387650512141, 0.3333333333333333703, 0.3170188387650512141, 0.3333333333333333703, 0.3170188387650512141, 0.3333333333333333703, 0.3170188387650512141, 0.3333333333333333703, 0.3170188387650512141, 0.3333333333333333703, 0.3170188387650512141, 0.3333333333333333703),
 ( 1.000000000000000000, 0.9510565162951535312, 1.000000000000000000, 0.9510565162951535312, 1.000000000000000000, 0.9510565162951535312, 1.000000000000000000, 0.9510565162951535312, 1.000000000000000000, 0.9510565162951535312, 1.000000000000000000, 0.9510565162951535312, 1.000000000000000000, 0.9510565162951535312, 1.000000000000000000, 0.9510565162951535312, 1.000000000000000000, 0.9510565162951535312, 1.000000000000000000, 0.9510565162951535312, 1.000000000000000000, 0.9510565162951535312, 1.000000000000000000, 0.9510565162951535312, 1.000000000000000000, 0.9510565162951535312, 1.000000000000000000, 0.9510565162951535312, 1.000000000000000000, 0.9510565162951535312, 1.000000000000000000, 0.9510565162951535312, 1.000000000000000000, 0.9510565162951535312, 1.000000000000000000, 0.9510565162951535312, 1.000000000000000000, 0.9510565162951535312, 1.000000000000000000, 0.9510565162951535312, 1.000000000000000000, 0.9510565162951535312, 1.000000000000000000, 0.9510565162951535312, 1.000000000000000000, 0.9510565162951535312, 1.000000000000000000, 0.9510565162951535312, 1.000000000000000000, 0.9510565162951535312, 1.000000000000000000, 0.9510565162951535312, 1.000000000000000000, 0.9510565162951535312, 1.000000000000000000, 0.9510565162951535312, 1.000000000000000000, 0.9510565162951535312, 1.000000000000000000, 0.9510565162951535312, 1.000000000000000000, 0.9510565162951535312, 1.000000000000000000, 0.9510565162951535312, 1.000000000000000000, 0.9510565162951535312, 1.000000000000000000, 0.9510565162951535312, 1.000000000000000000, 0.9510565162951535312, 1.000000000000000000, 0.9510565162951535312, 1.000000000000000000, 0.9510565162951535312, 1.000000000000000000, 0.9510565162951535312, 1.000000000000000000, 0.9510565162951535312, 1.000000000000000000, 0.9510565162951535312, 1.000000000000000000, 0.9510565162951535312, 1.000000000000000000, 0.9510565162951535312, 1.000000000000000000, 0.9510565162951535312, 1.000000000000000000, 0.9510565162951535312, 1.000000000000000000, 0.9510565162951535312, 1.000000000000000000, 0.9510565162951535312, 1.000000000000000000, 0.9510565162951535312, 1.000000000000000000, 0.9510565162951535312, 1.000000000000000000, 0.9510565162951535312, 1.000000000000000000, 0.9510565162951535312, 1.000000000000000000),
 ( 0.3333333333333333703, 0.3170188387650512141, 0.3333333333333333703, 0.3170188387650512141, 0.3333333333333333703, 0.3170188387650512141, 0.3333333333333333703, 0.3170188387650512141, 0.3333333333333333703, 0.3170188387650512141, 0.3333333333333333703, 0.3170188387650512141, 0.3333333333333333703, 0.3170188387650512141, 0.3333333333333333703, 0.3170188387650512141, 0.3333333333333333703, 0.3170188387650512141, 0.3333333333333333703, 0.3170188387650512141, 0.3333333333333333703, 0.3170188387650512141, 0.3333333333333333703, 0.3170188387650512141, 0.3333333333333333703, 0.3170188387650512141, 0.3333333333333333703, 0.3170188387650512141, 0.3333333333333333703, 0.3170188387650512141, 0.3333333333333333703, 0.3170188387650512141, 0.3333333333333333703, 0.3170188387650512141, 0.3333333333333333703, 0.3170188387650512141, 0.3333333333333333703, 0.3170188387650512141, 0.3333333333333333703, 0.3170188387650512141, 0.3333333333333333703, 0.3170188387650512141, 0.3333333333333333703, 0.3170188387650512141, 0.3333333333333333703, 0.3170188387650512141, 0.3333333333333333703, 0.3170188387650512141, 0.3333333333333333703, 0.3170188387650512141, 0.3333333333333333703, 0.3170188387650512141, 0.3333333333333333703, 0.3170188387650512141, 0.3333333333333333703, 0.3170188387650512141, 0.3333333333333333703, 0.3170188387650512141, 0.3333333333333333703, 0.3170188387650512141, 0.3333333333333333703, 0.3170188387650512141, 0.3333333333333333703, 0.3170188387650512141, 0.3333333333333333703, 0.3170188387650512141, 0.3333333333333333703, 0.3170188387650512141, 0.3333333333333333703, 0.3170188387650512141, 0.3333333333333333703, 0.3170188387650512141, 0.3333333333333333703, 0.3170188387650512141, 0.3333333333333333703, 0.3170188387650512141, 0.3333333333333333703, 0.3170188387650512141, 0.3333333333333333703, 0.3170188387650512141, 0.3333333333333333703, 0.3170188387650512141, 0.3333333333333333703, 0.3170188387650512141, 0.3333333333333333703, 0.3170188387650512141, 0.3333333333333333703, 0.3170188387650512141, 0.3333333333333333703, 0.3170188387650512141, 0.3333333333333333703, 0.3170188387650512141, 0.3333333333333333703, 0.3170188387650512141, 0.3333333333333333703, 0.3170188387650512141, 0.3333333333333333703, 0.3170188387650512141, 0.3333333333333333703, 0.3170188387650512141, 0.3333333333333333703),
 ( 0.3333333333333333703, 0.3170188387650512141, 0.3333333333333333703, 0.3170188387650512141, 0.3333333333333333703, 0.3170188387650512141, 0.3333333333333333703, 0.3170188387650512141, 0.3333333333333333703, 0.3170188387650512141, 0.3333333333333333703, 0.3170188387650512141, 0.3333333333333333703, 0.3170188387650512141, 0.3333333333333333703, 0.3170188387650512141, 0.3333333333333333703, 0.3170188387650512141, 0.3333333333333333703, 0.3170188387650512141, 0.3333333333333333703, 0.3170188387650512141, 0.3333333333333333703, 0.3170188387650512141, 0.3333333333333333703, 0.3170188387650512141, 0.3333333333333333703, 0.3170188387650512141, 0.3333333333333333703, 0.3170188387650512141, 0.3333333333333333703, 0.3170188387650512141, 0.3333333333333333703, 0.3170188387650512141, 0.3333333333333333703, 0.3170188387650512141, 0.3333333333333333703, 0.3170188387650512141, 0.3333333333333333703, 0.3170188387650512141, 0.3333333333333333703, 0.3170188387650512141, 0.3333333333333333703, 0.3170188387650512141, 0.3333333333333333703, 0.3170188387650512141, 0.3333333333333333703, 0.3170188387650512141, 0.3333333333333333703, 0.3170188387650512141, 0.3333333333333333703, 0.3170188387650512141, 0.3333333333333333703, 0.3170188387650512141, 0.3333333333333333703, 0.3170188387650512141, 0.3333333333333333703, 0.3170188387650512141, 0.3333333333333333703, 0.3170188387650512141, 0.3333333333333333703, 0.3170188387650512141, 0.3333333333333333703, 0.3170188387650512141, 0.3333333333333333703, 0.3170188387650512141, 0.3333333333333333703, 0.3170188387650512141, 0.3333333333333333703, 0.3170188387650512141, 0.3333333333333333703, 0.3170188387650512141, 0.3333333333333333703, 0.3170188387650512141, 0.3333333333333333703, 0.3170188387650512141, 0.3333333333333333703, 0.3170188387650512141, 0.3333333333333333703, 0.3170188387650512141, 0.3333333333333333703, 0.3170188387650512141, 0.3333333333333333703, 0.3170188387650512141, 0.3333333333333333703, 0.3170188387650512141, 0.3333333333333333703, 0.3170188387650512141, 0.3333333333333333703, 0.3170188387650512141, 0.3333333333333333703, 0.3170188387650512141, 0.3333333333333333703, 0.3170188387650512141, 0.3333333333333333703, 0.3170188387650512141, 0.3333333333333333703, 0.3170188387650512141, 0.3333333333333333703, 0.3170188387650512141, 0.3333333333333333703),
 ( 1.000000000000000000, 0.9510565162951535312, 1.000000000000000000, 0.9510565162951535312, 1.000000000000000000, 0.9510565162951535312, 1.000000000000000000, 0.9510565162951535312, 1.000000000000000000, 0.9510565162951535312, 1.000000000000000000, 0.9510565162951535312, 1.000000000000000000, 0.9510565162951535312, 1.000000000000000000, 0.9510565162951535312, 1.000000000000000000, 0.9510565162951535312, 1.000000000000000000, 0.9510565162951535312, 1.000000000000000000, 0.9510565162951535312, 1.000000000000000000, 0.9510565162951535312, 1.000000000000000000, 0.9510565162951535312, 1.000000000000000000, 0.9510565162951535312, 1.000000000000000000, 0.9510565162951535312, 1.000000000000000000, 0.9510565162951535312, 1.000000000000000000, 0.9510565162951535312, 1.000000000000000000, 0.9510565162951535312, 1.000000000000000000, 0.9510565162951535312, 1.000000000000000000, 0.9510565162951535312, 1.000000000000000000, 0.9510565162951535312, 1.000000000000000000, 0.9510565162951535312, 1.000000000000000000, 0.9510565162951535312, 1.000000000000000000, 0.9510565162951535312, 1.000000000000000000, 0.9510565162951535312, 1.000000000000000000, 0.9510565162951535312, 1.000000000000000000, 0.9510565162951535312, 1.000000000000000000, 0.9510565162951535312, 1.000000000000000000, 0.9510565162951535312, 1.000000000000000000, 0.9510565162951535312, 1.000000000000000000, 0.9510565162951535312, 1.000000000000000000, 0.9510565162951535312, 1.000000000000000000, 0.9510565162951535312, 1.000000000000000000, 0.9510565162951535312, 1.000000000000000000, 0.9510565162951535312, 1.000000000000000000, 0.9510565162951535312, 1.000000000000000000, 0.9510565162951535312, 1.000000000000000000, 0.9510565162951535312, 1.000000000000000000, 0.9510565162951535312, 1.000000000000000000, 0.9510565162951535312, 1.000000000000000000, 0.9510565162951535312, 1.000000000000000000, 0.9510565162951535312, 1.000000000000000000, 0.9510565162951535312, 1.000000000000000000, 0.9510565162951535312, 1.000000000000000000, 0.9510565162951535312, 1.000000000000000000, 0.9510565162951535312, 1.000000000000000000, 0.9510565162951535312, 1.000000000000000000, 0.9510565162951535312, 1.000000000000000000, 0.9510565162951535312, 1.000000000000000000, 0.9510565162951535312, 1.000000000000000000) ) ) 
 REPRESENTATION_ITEM ( '' )  SURFACE ( )  );
#5423=CARTESIAN_POINT ( 'NONE',  ( -2.042957248827969252, 4.009529358847651714, 13.43999999999999950 ) ) ;
#5435=CARTESIAN_POINT ( 'NONE',  ( 4.155232146225751322, -4.023224611898307934, 12.89605171672202211 ) ) ;
#5438=CARTESIAN_POINT ( 'NONE',  ( 5.110351332421769754, 2.708615832122969191, 12.33605171672202339 ) ) ;
#5446=CARTESIAN_POINT ( 'NONE',  ( 3.951860609387084722, 3.826313983664940022, 4.603948283277976117 ) ) ;
#5459=CARTESIAN_POINT ( 'NONE',  ( 0.7401821875142697849, -4.673326407553650697, 9.379999999999995453 ) ) ;
#5461=CARTESIAN_POINT ( 'NONE',  ( 0.8124729078102063129, -5.726445515403652209, 11.18394828327797441 ) ) ;
#5474=CARTESIAN_POINT ( 'NONE',  ( 3.345732310141667387, -3.345732310141653620, 11.90000000000000036 ) ) ;
#5483=CARTESIAN_POINT ( 'NONE',  ( 5.726445515403654873, -0.8124729078101852187, 9.816051716722022036 ) ) ;
#5489=CARTESIAN_POINT ( 'NONE',  ( 4.430710083317573655, 0.7916369971161595354, 1.276051716722023333 ) ) ;
#5498=CARTESIAN_POINT ( 'NONE',  ( -5.195105386651219348, -2.542276634908102295, 8.943948283277975975 ) ) ;
#5512=CARTESIAN_POINT ( 'NONE',  ( 2.148092372876330369, 4.215868657802593233, 11.05999999999999872 ) ) ;
#5513=EDGE_CURVE ( 'NONE', #2194, #8250, #1088, .T. ) ;
#5516=CARTESIAN_POINT ( 'NONE',  ( -5.446173322633801384, -0.7727076532861678615, 11.88394828327797548 ) ) ;
#5530=CARTESIAN_POINT ( 'NONE',  ( -3.345732310141667831, 3.345732310141653620, 7.699999999999998401 ) ) ;
#5536=CARTESIAN_POINT ( 'NONE',  ( -4.687928535947287756, 0.6479879772514611780, 5.616051716722022746 ) ) ;
#5541=CARTESIAN_POINT ( 'NONE',  ( -5.110351332421769754, -2.708615832122969191, 13.73605171672202019 ) ) ;
#5543=( NAMED_UNIT ( * ) SI_UNIT ( $, .STERADIAN. ) SOLID_ANGLE_UNIT ( ) );
#5550=CARTESIAN_POINT ( 'NONE',  ( -0.8124729078102072011, 5.726445515403652209, 4.183948283277976188 ) ) ;
#5562=CARTESIAN_POINT ( 'NONE',  ( -4.009529358847660596, 2.042957248827953265, 7.559999999999998721 ) ) ;
#5565=CARTESIAN_POINT ( 'NONE',  ( -4.023224611898323033, 4.155232146225737111, 6.703948283277976650 ) ) ;
#5569=CARTESIAN_POINT ( 'NONE',  ( -4.900535883036028828, 2.496947748567499126, 1.959999999999999964 ) ) ;
#5578=CARTESIAN_POINT ( 'NONE',  ( 2.042957248827968808, -4.009529358847652603, 12.03999999999999915 ) ) ;
#5587=SURFACE_SIDE_STYLE ('',( #3052 ) ) ;
#5595=CARTESIAN_POINT ( 'NONE',  ( 3.119207202478379681, 3.244753828200549695, 0.9960517167220231949 ) ) ;
#5605=CARTESIAN_POINT ( 'NONE',  ( -2.496947748567517333, 4.900535883036019058, 7.839999999999999858 ) ) ;
#5607=CARTESIAN_POINT ( 'NONE',  ( 5.711843387010018702, -0.9046671180729751738, 3.219999999999999751 ) ) ;
#5610=DIRECTION ( 'NONE',  ( 0.000000000000000000, 0.000000000000000000, 1.000000000000000000 ) ) ;
#5617=CARTESIAN_POINT ( 'NONE',  ( 2.148092372876330369, 4.215868657802593233, 5.459999999999997300 ) ) ;
#5620=CARTESIAN_POINT ( 'NONE',  ( 4.089228379062037178, -4.089228379062022967, 6.299999999999999822 ) ) ;
#5623=CARTESIAN_POINT ( 'NONE',  ( -3.889087296526005044, -3.889087296526019255, 1.399999999999999689 ) ) ;
#5632=CARTESIAN_POINT ( 'NONE',  ( -4.258245684917310925, -2.064922774268914019, 0.5439482832779766186 ) ) ;
#5641=CARTESIAN_POINT ( 'NONE',  ( -3.345732310141667831, 3.345732310141653620, 2.099999999999999645 ) ) ;
#5646=CARTESIAN_POINT ( 'NONE',  ( 4.173491630687861331, 2.231261971483781359, 3.936051716722023031 ) ) ;
#5654=CARTESIAN_POINT ( 'NONE',  ( 4.900535883036028828, -2.496947748567499126, 3.359999999999999876 ) ) ;
#5656=CARTESIAN_POINT ( 'NONE',  ( 0.9480714621563713917, 5.418398423912717199, 12.72394828327797711 ) ) ;
#5665=CARTESIAN_POINT ( 'NONE',  ( 3.279728542977952799, -3.411736077305369541, 2.503948283277976472 ) ) ;
#5668=CARTESIAN_POINT ( 'NONE',  ( -0.9046671180729963790, 5.711843387010016926, 7.979999999999999538 ) ) ;
#5673=CARTESIAN_POINT ( 'NONE',  ( 5.432285873273257515, 0.8603895577212793411, 3.079999999999999627 ) ) ;
#5682=CARTESIAN_POINT ( 'NONE',  ( 4.258245684917310037, 2.064922774268912686, 4.743948283277974909 ) ) ;
#5690=CARTESIAN_POINT ( 'NONE',  ( -2.042957248827969252, 4.009529358847651714, 5.039999999999999147 ) ) ;
#5693=CARTESIAN_POINT ( 'NONE',  ( -2.064922774268895811, -4.258245684917318918, 10.65605171672202012 ) ) ;
#5700=CARTESIAN_POINT ( 'NONE',  ( -4.900535883036028828, 2.496947748567499126, 1.959999999999999964 ) ) ;
#5702=CARTESIAN_POINT ( 'NONE',  ( 5.152728359536493663, 2.625446233515533745, 0.1399999999999999856 ) ) ;
#5714=CARTESIAN_POINT ( 'NONE',  ( -4.258245684917310925, -2.064922774268914019, 3.343948283277975886 ) ) ;
#5717=CARTESIAN_POINT ( 'NONE',  ( 0.9046671180729951578, -5.711843387010016926, 0.9799999999999997602 ) ) ;
#5726=CARTESIAN_POINT ( 'NONE',  ( -0.6162731882459178134, -4.458484982038665834, 4.916051716722023457 ) ) ;
#5728=CARTESIAN_POINT ( 'NONE',  ( 3.969226411068985882, -2.122056237541205981, 7.963948283277976437 ) ) ;
#5741=CARTESIAN_POINT ( 'NONE',  ( -4.215868657802586128, -2.148092372876348133, 4.339999999999999858 ) ) ;
#5745=CARTESIAN_POINT ( 'NONE',  ( -0.8323763977770610722, 4.658724279160015413, 11.77605171672202289 ) ) ;
#5755=CARTESIAN_POINT ( 'NONE',  ( -2.496947748567517333, 4.900535883036019058, 5.039999999999999147 ) ) ;
#5756=CARTESIAN_POINT ( 'NONE',  ( -3.889087296526005044, -3.889087296526019255, 6.999999999999999112 ) ) ;
#5757=CARTESIAN_POINT ( 'NONE',  ( 3.951860609387084722, 3.826313983664940022, 10.20394828327797399 ) ) ;
#5769=CARTESIAN_POINT ( 'NONE',  ( -4.258245684917310925, -2.064922774268914019, 0.5439482832779766186 ) ) ;
#5774=CARTESIAN_POINT ( 'NONE',  ( 2.625446233515515537, 5.152728359536502545, 2.659999999999998366 ) ) ;
#5776=CARTESIAN_POINT ( 'NONE',  ( 5.152728359536493663, 2.625446233515533745, 11.33999999999999808 ) ) ;
#5781=CARTESIAN_POINT ( 'NONE',  ( -4.430710083317573655, -0.7916369971161599794, 5.476051716722023066 ) ) ;
#5784=CARTESIAN_POINT ( 'NONE',  ( -4.258245684917310925, -2.064922774268914019, 8.943948283277975975 ) ) ;
#5787=CARTESIAN_POINT ( 'NONE',  ( -4.940838830814703542, 2.417848759854245078, 8.556051716722022249 ) ) ;
#5792=CARTESIAN_POINT ( 'NONE',  ( -4.009529358847660596, 2.042957248827953265, 4.759999999999999787 ) ) ;
#5796=CARTESIAN_POINT ( 'NONE',  ( 3.411736077305382420, -3.279728542977940364, 10.09605171672202140 ) ) ;
#5805=CARTESIAN_POINT ( 'NONE',  ( -0.8603895577212598011, -5.432285873273260179, 3.919999999999999929 ) ) ;
#5806=CARTESIAN_POINT ( 'NONE',  ( -2.625446233515515981, -5.152728359536500768, 4.059999999999999609 ) ) ;
#5807=CARTESIAN_POINT ( 'NONE',  ( 3.889087296526005488, 3.889087296526018811, 2.799999999999999378 ) ) ;
#5822=CARTESIAN_POINT ( 'NONE',  ( 3.181980515339458471, 3.181980515339470461, 13.99999999999999822 ) ) ;
#5825=CARTESIAN_POINT ( 'NONE',  ( -2.496947748567517333, 4.900535883036019058, 2.239999999999999769 ) ) ;
#5828=CARTESIAN_POINT ( 'NONE',  ( -5.711843387010019590, 0.9046671180729746187, 7.419999999999999041 ) ) ;
#5834=CARTESIAN_POINT ( 'NONE',  ( -2.064922774268895811, -4.258245684917318918, 2.256051716722022871 ) ) ;
#5837=CARTESIAN_POINT ( 'NONE',  ( -4.258245684917310925, -2.064922774268914019, 3.343948283277975886 ) ) ;
#5840=CARTESIAN_POINT ( 'NONE',  ( 2.542276634908080535, 5.195105386651229118, 3.656051716722022782 ) ) ;
#5849=CARTESIAN_POINT ( 'NONE',  ( 0.8323763977770604061, -4.658724279160015413, 4.776051716722021112 ) ) ;
#5857=CARTESIAN_POINT ( 'NONE',  ( -3.889087296526005044, -3.889087296526019255, 9.799999999999998934 ) ) ;
#5858=CARTESIAN_POINT ( 'NONE',  ( -4.900535883036028828, 2.496947748567499126, 7.559999999999998721 ) ) ;
#5859=CARTESIAN_POINT ( 'NONE',  ( 4.900535883036028828, -2.496947748567499126, 11.75999999999999979 ) ) ;
#5871=CARTESIAN_POINT ( 'NONE',  ( -4.673326407553653361, 0.7401821875142517992, 13.01999999999999424 ) ) ;
#5877=CARTESIAN_POINT ( 'NONE',  ( -0.8603895577212598011, -5.432285873273260179, 3.919999999999999929 ) ) ;
#5881=CARTESIAN_POINT ( 'NONE',  ( -4.430710083317573655, -0.7916369971161599794, 2.676051716722023244 ) ) ;
#5883=CARTESIAN_POINT ( 'NONE',  ( 4.458484982038663169, 0.6162731882459350219, 4.883948283277976365 ) ) ;
#5887=CARTESIAN_POINT ( 'NONE',  ( -5.418398423912711870, -0.9480714621563917088, 5.476051716722023066 ) ) ;
#5891=CARTESIAN_POINT ( 'NONE',  ( 2.148092372876330369, 4.215868657802594122, 13.85999999999999943 ) ) ;
#5894=CARTESIAN_POINT ( 'NONE',  ( 2.064922774268895811, 4.258245684917319807, 12.05605171672202047 ) ) ;
#5907=CARTESIAN_POINT ( 'NONE',  ( -0.9046671180729963790, 5.711843387010016926, 13.57999999999999474 ) ) ;
#5908=CARTESIAN_POINT ( 'NONE',  ( 2.496947748567516889, -4.900535883036019946, 3.639999999999999680 ) ) ;
#5909=CARTESIAN_POINT ( 'NONE',  ( 5.432285873273257515, 0.8603895577212793411, 8.679999999999997939 ) ) ;
#5921=CARTESIAN_POINT ( 'NONE',  ( 3.244753828200538148, 3.119207202478391672, 7.403948283277976827 ) ) ;
#5926=CARTESIAN_POINT ( 'NONE',  ( -0.9046671180729963790, 5.711843387010016926, 13.57999999999999474 ) ) ;
#5929=CARTESIAN_POINT ( 'NONE',  ( -0.9046671180729962680, 5.711843387010016926, 7.979999999999999538 ) ) ;
#5935=CARTESIAN_POINT ( 'NONE',  ( -0.6162731882459178134, -4.458484982038665834, 13.31605171672202204 ) ) ;
#5937=CARTESIAN_POINT ( 'NONE',  ( 4.023224611898322145, -4.155232146225737111, 2.503948283277976472 ) ) ;
#5940=CARTESIAN_POINT ( 'NONE',  ( -3.826313983664925811, -3.951860609387098489, 2.396051716722022551 ) ) ;
#5945=CARTESIAN_POINT ( 'NONE',  ( -0.7039550926810301812, -4.444597532678121965, 6.719999999999999751 ) ) ;
#5946=CARTESIAN_POINT ( 'NONE',  ( -4.673326407553653361, 0.7401821875142517992, 4.620000000000000107 ) ) ;
#5955=CARTESIAN_POINT ( 'NONE',  ( -4.900535883036028828, 2.496947748567499126, 10.35999999999999943 ) ) ;
#5957=CARTESIAN_POINT ( 'NONE',  ( 0.9046671180729951578, -5.711843387010016926, 3.779999999999998472 ) ) ;
#5958=CARTESIAN_POINT ( 'NONE',  ( -4.089228379062038066, 4.089228379062021190, 7.699999999999998401 ) ) ;
#5972=CARTESIAN_POINT ( 'NONE',  ( 4.658724279160018966, -0.8323763977770426425, 10.62394828327797569 ) ) ;
#5978=CARTESIAN_POINT ( 'NONE',  ( 0.8603895577212593571, 5.432285873273261068, 8.119999999999999218 ) ) ;
#5982=CARTESIAN_POINT ( 'NONE',  ( -4.430710083317573655, -0.7916369971161599794, 13.87605171672202253 ) ) ;
#5985=CARTESIAN_POINT ( 'NONE',  ( -0.6479879772514802738, 4.687928535947285091, 12.58394828327797477 ) ) ;
#5988=APPLICATION_CONTEXT ( 'automotive_design' ) ;
#5990=CARTESIAN_POINT ( 'NONE',  ( -4.155232146225753098, 4.023224611898306158, 8.696051716722022817 ) ) ;
#5995=CARTESIAN_POINT ( 'NONE',  ( 3.345732310141667387, -3.345732310141654064, 9.099999999999996092 ) ) ;
#5998=CARTESIAN_POINT ( 'NONE',  ( 3.181980515339458471, 3.181980515339470461, 2.799999999999999378 ) ) ;
#6009=CARTESIAN_POINT ( 'NONE',  ( -2.625446233515515981, -5.152728359536500768, 9.659999999999994813 ) ) ;
#6010=CARTESIAN_POINT ( 'NONE',  ( -5.711843387010018702, 0.9046671180729746187, 10.21999999999999709 ) ) ;
#6011=CARTESIAN_POINT ( 'NONE',  ( -0.8603895577212598011, -5.432285873273260179, 12.31999999999999851 ) ) ;
#6025=CARTESIAN_POINT ( 'NONE',  ( 0.8124729078102063129, -5.726445515403652209, -0.01605171672202330979 ) ) ;
#6035=CARTESIAN_POINT ( 'NONE',  ( 0.8323763977770604061, -4.658724279160015413, 13.17605171672201969 ) ) ;
#6037=CARTESIAN_POINT ( 'NONE',  ( -2.708615832122950096, -5.110351332421780413, 3.063948283277976081 ) ) ;
#6046=CARTESIAN_POINT ( 'NONE',  ( 0.7401821875142697849, -4.673326407553650697, 6.579999999999999183 ) ) ;
#6048=CARTESIAN_POINT ( 'NONE',  ( 4.444597532678119300, 0.7039550926810472786, 5.879999999999999893 ) ) ;
#6058=CARTESIAN_POINT ( 'NONE',  ( 3.889087296526005488, 3.889087296526018811, 13.99999999999999822 ) ) ;
#6060=CARTESIAN_POINT ( 'NONE',  ( -5.432285873273256627, -0.8603895577212797852, 12.87999999999999901 ) ) ;
#6061=CARTESIAN_POINT ( 'NONE',  ( -5.152728359536494551, -2.625446233515535077, 9.939999999999994174 ) ) ;
#6078=CARTESIAN_POINT ( 'NONE',  ( 4.458484982038663169, 0.6162731882459350219, 10.48394828327797512 ) ) ;
#6084=CARTESIAN_POINT ( 'NONE',  ( -5.432285873273256627, -0.8603895577212797852, 12.87999999999999901 ) ) ;
#6092=CARTESIAN_POINT ( 'NONE',  ( -4.049832306626335310, 1.963858260114700327, 14.15605171672202012 ) ) ;
#6098=CARTESIAN_POINT ( 'NONE',  ( 5.446173322633801384, 0.7727076532861675284, 2.083948283277976543 ) ) ;
#6109=CARTESIAN_POINT ( 'NONE',  ( 0.7039550926810297371, 4.444597532678122853, 13.71999999999999886 ) ) ;
#6110=CARTESIAN_POINT ( 'NONE',  ( -4.687928535947287756, 0.6479879772514611780, 14.01605171672202310 ) ) ;
#6118=CARTESIAN_POINT ( 'NONE',  ( -5.418398423912711870, -0.9480714621563917088, 5.476051716722023066 ) ) ;
#6119=CARTESIAN_POINT ( 'NONE',  ( 4.089228379062037178, -4.089228379062022967, 11.90000000000000036 ) ) ;
#6132=CARTESIAN_POINT ( 'NONE',  ( -4.258245684917310925, -2.064922774268914019, 8.943948283277975975 ) ) ;
#6146=CARTESIAN_POINT ( 'NONE',  ( 4.673326407553653361, -0.7401821875142523544, 0.4199999999999999845 ) ) ;
#6148=CARTESIAN_POINT ( 'NONE',  ( 5.446173322633801384, 0.7727076532861675284, -0.7160517167220232793 ) ) ;
#6161=CARTESIAN_POINT ( 'NONE',  ( 4.009529358847659708, -2.042957248827953709, 0.5599999999999999423 ) ) ;
#6163=MECHANICAL_DESIGN_GEOMETRIC_PRESENTATION_REPRESENTATION('',(#259),#4138);
#6171=CARTESIAN_POINT ( 'NONE',  ( 0.7727076532861471003, 5.446173322633805824, 9.116051716722020970 ) ) ;
#6187=CARTESIAN_POINT ( 'NONE',  ( -5.697241258616385196, 0.9968613283357647958, 6.423948283277978177 ) ) ;
#6199=CARTESIAN_POINT ( 'NONE',  ( 4.444597532678119300, 0.7039550926810472786, 3.079999999999999627 ) ) ;
#6202=CARTESIAN_POINT ( 'NONE',  ( -4.023224611898323033, 4.155232146225737111, 9.503948283277974696 ) ) ;
#6211=CARTESIAN_POINT ( 'NONE',  ( -4.673326407553653361, 0.7401821875142517992, 10.21999999999999709 ) ) ;
#6219=CARTESIAN_POINT ( 'NONE',  ( 2.542276634908080535, 5.195105386651229118, 6.456051716722022604 ) ) ;
#6234=CARTESIAN_POINT ( 'NONE',  ( -0.8124729078102072011, 5.726445515403652209, 1.383948283277976365 ) ) ;
#6238=AXIS2_PLACEMENT_3D ( 'NONE', #8191, #4149, #7229 ) ;
#6248=CARTESIAN_POINT ( 'NONE',  ( -4.215868657802586128, -2.148092372876348133, 9.939999999999994174 ) ) ;
#6251=CARTESIAN_POINT ( 'NONE',  ( -5.195105386651219348, -2.542276634908102295, 6.143948283277977040 ) ) ;
#6265=CARTESIAN_POINT ( 'NONE',  ( -2.042957248827969252, 4.009529358847651714, 10.63999999999999879 ) ) ;
#6275=SURFACE_STYLE_USAGE ( .BOTH. , #5587 ) ;
#6277=CARTESIAN_POINT ( 'NONE',  ( 5.418398423912711870, 0.9480714621563913758, 9.676051716722021467 ) ) ;
#6282=CARTESIAN_POINT ( 'NONE',  ( 4.155232146225751322, -4.023224611898307934, 12.89605171672202211 ) ) ;
#6290=CARTESIAN_POINT ( 'NONE',  ( 0.9480714621563713917, 5.418398423912717199, 1.523948283277976268 ) ) ;
#6302=CARTESIAN_POINT ( 'NONE',  ( -0.7039550926810301812, -4.444597532678121965, 9.519999999999999574 ) ) ;
#6304=CARTESIAN_POINT ( 'NONE',  ( 4.023224611898322145, -4.155232146225737111, 8.103948283277974340 ) ) ;
#6317=CARTESIAN_POINT ( 'NONE',  ( -3.345732310141667831, 3.345732310141653620, 10.50000000000000000 ) ) ;
#6328=CARTESIAN_POINT ( 'NONE',  ( -3.826313983664925811, -3.951860609387098489, 5.196051716722022817 ) ) ;
#6333=CARTESIAN_POINT ( 'NONE',  ( 3.411736077305382420, -3.279728542977940364, 1.696051716722023484 ) ) ;
#6336=( NAMED_UNIT ( * ) SI_UNIT ( $, .STERADIAN. ) SOLID_ANGLE_UNIT ( ) );
#6346=CARTESIAN_POINT ( 'NONE',  ( -3.951860609387083834, -3.826313983664940466, 6.003948283277975584 ) ) ;
#6361=CARTESIAN_POINT ( 'NONE',  ( -4.673326407553653361, 0.7401821875142517992, 10.21999999999999709 ) ) ;
#6364=CARTESIAN_POINT ( 'NONE',  ( 5.432285873273257515, 0.8603895577212793411, 0.2799999999999999156 ) ) ;
#6378=CARTESIAN_POINT ( 'NONE',  ( -4.444597532678119300, -0.7039550926810477227, 10.07999999999999829 ) ) ;
#6388=CARTESIAN_POINT ( 'NONE',  ( -0.8323763977770610722, 4.658724279160015413, 3.376051716722022977 ) ) ;
#6394=CARTESIAN_POINT ( 'NONE',  ( -5.432285873273256627, -0.8603895577212797852, 7.279999999999999361 ) ) ;
#6397=CARTESIAN_POINT ( 'NONE',  ( 5.195105386651219348, 2.542276634908100075, 4.743948283277974909 ) ) ;
#6407=CARTESIAN_POINT ( 'NONE',  ( -3.345732310141667831, 3.345732310141653620, 7.699999999999998401 ) ) ;
#6412=CARTESIAN_POINT ( 'NONE',  ( -5.697241258616385196, 0.9968613283357647958, 6.423948283277978177 ) ) ;
#6417=EDGE_CURVE ( 'NONE', #2194, #5388, #7713, .T. ) ;
#6426=CARTESIAN_POINT ( 'NONE',  ( 4.258245684917310037, 2.064922774268912686, -0.8560517167220232926 ) ) ;
#6438=CARTESIAN_POINT ( 'NONE',  ( 4.215868657802586128, 2.148092372876346801, 0.1400000000000000411 ) ) ;
#6442=CARTESIAN_POINT ( 'NONE',  ( 4.940838830814703542, -2.417848759854246410, 12.75605171672202331 ) ) ;
#6451=CARTESIAN_POINT ( 'NONE',  ( 5.432285873273257515, 0.8603895577212793411, 3.079999999999999627 ) ) ;
#6453=CARTESIAN_POINT ( 'NONE',  ( -4.023224611898323033, 4.155232146225737111, 9.503948283277974696 ) ) ;
#6462=PLANE ( 'NONE',  #8954 ) ;
#6463=CARTESIAN_POINT ( 'NONE',  ( -0.7401821875142701179, 4.673326407553649808, 13.57999999999999474 ) ) ;
#6466=CARTESIAN_POINT ( 'NONE',  ( -0.9046671180729963790, 5.711843387010016926, 2.379999999999999893 ) ) ;
#6470=CARTESIAN_POINT ( 'NONE',  ( 5.432285873273257515, 0.8603895577212793411, 0.2799999999999999156 ) ) ;
#6478=CARTESIAN_POINT ( 'NONE',  ( 0.7916369971161419938, 4.430710083317576320, 1.523948283277976268 ) ) ;
#6489=CARTESIAN_POINT ( 'NONE',  ( -0.7039550926810301812, -4.444597532678121965, 3.919999999999999929 ) ) ;
#6492=CARTESIAN_POINT ( 'NONE',  ( 4.155232146225751322, -4.023224611898307934, 10.09605171672202140 ) ) ;
#6500=CARTESIAN_POINT ( 'NONE',  ( -5.152728359536494551, -2.625446233515535077, 1.540000000000000036 ) ) ;
#6503=CARTESIAN_POINT ( 'NONE',  ( 5.432285873273257515, 0.8603895577212793411, 3.079999999999999627 ) ) ;
#6515=DIRECTION ( 'NONE',  ( -0.7043149233066458015, 0.7043149233066440251, -0.08877487040322762368 ) ) ;
#6516=CARTESIAN_POINT ( 'NONE',  ( 4.458484982038663169, 0.6162731882459350219, 2.083948283277976543 ) ) ;
#6519=CARTESIAN_POINT ( 'NONE',  ( -0.8603895577212598011, -5.432285873273260179, 3.919999999999999929 ) ) ;
#6530=CARTESIAN_POINT ( 'NONE',  ( -4.173491630687863108, -2.231261971483782691, 2.536051716722023119 ) ) ;
#6536=CARTESIAN_POINT ( 'NONE',  ( 3.969226411068985882, -2.122056237541205981, 5.163948283277975726 ) ) ;
#6543=CARTESIAN_POINT ( 'NONE',  ( 4.215868657802586128, 2.148092372876346801, 2.939999999999999503 ) ) ;
#6546=CARTESIAN_POINT ( 'NONE',  ( 4.049832306626335310, -1.963858260114701215, 9.956051716722022604 ) ) ;
#6554=CARTESIAN_POINT ( 'NONE',  ( 0.8603895577212593571, 5.432285873273261068, 2.519999999999999574 ) ) ;
#6556=CARTESIAN_POINT ( 'NONE',  ( 3.889087296526005488, 3.889087296526018811, 5.599999999999998757 ) ) ;
#6557=CARTESIAN_POINT ( 'NONE',  ( 5.152728359536493663, 2.625446233515533745, 2.939999999999999059 ) ) ;
#6569=CARTESIAN_POINT ( 'NONE',  ( -3.969226411068985882, 2.122056237541205537, 0.9639482832779766586 ) ) ;
#6572=CARTESIAN_POINT ( 'NONE',  ( 3.889087296526005488, 3.889087296526018811, 2.799999999999999378 ) ) ;
#6574=CARTESIAN_POINT ( 'NONE',  ( -5.711843387010019590, 0.9046671180729746187, 10.21999999999999886 ) ) ;
#6580=CARTESIAN_POINT ( 'NONE',  ( -2.064922774268895811, -4.258245684917318918, 5.056051716722023137 ) ) ;
#6582=CARTESIAN_POINT ( 'NONE',  ( -1.963858260114716980, 4.049832306626327316, 6.843948283277976330 ) ) ;
#6586=CARTESIAN_POINT ( 'NONE',  ( 5.418398423912711870, 0.9480714621563913758, 4.076051716722022711 ) ) ;
#6597=CARTESIAN_POINT ( 'NONE',  ( 2.064922774268895811, 4.258245684917319807, 9.256051716722023315 ) ) ;
#6607=CARTESIAN_POINT ( 'NONE',  ( -2.496947748567517333, 4.900535883036019058, 2.239999999999999769 ) ) ;
#6608=CARTESIAN_POINT ( 'NONE',  ( 2.496947748567516889, -4.900535883036019946, 6.439999999999999503 ) ) ;
#6610=CARTESIAN_POINT ( 'NONE',  ( -4.860232935257354114, 2.576046737280751842, 12.16394828327797661 ) ) ;
#6625=CARTESIAN_POINT ( 'NONE',  ( 3.345732310141667387, -3.345732310141653620, 11.90000000000000036 ) ) ;
#6628=CARTESIAN_POINT ( 'NONE',  ( -5.711843387010018702, 0.9046671180729746187, 7.419999999999998153 ) ) ;
#6631=CARTESIAN_POINT ( 'NONE',  ( -3.889087296526005044, -3.889087296526019255, 4.200000000000000178 ) ) ;
#6635=CARTESIAN_POINT ( 'NONE',  ( -4.430710083317573655, -0.7916369971161599794, 8.276051716722021112 ) ) ;
#6637=CARTESIAN_POINT ( 'NONE',  ( 2.231261971483764484, 4.173491630687871101, 7.263948283277976259 ) ) ;
#6640=CARTESIAN_POINT ( 'NONE',  ( -2.576046737280769605, 4.860232935257343456, 3.236051716722023297 ) ) ;
#6644=CARTESIAN_POINT ( 'NONE',  ( 3.181980515339458471, 3.181980515339470461, 2.799999999999999378 ) ) ;
#6647=CARTESIAN_POINT ( 'NONE',  ( 4.687928535947288644, -0.6479879772514620662, 12.61605171672202097 ) ) ;
#6655=CARTESIAN_POINT ( 'NONE',  ( -4.155232146225753098, 4.023224611898306158, 3.096051716722023617 ) ) ;
#6656=CARTESIAN_POINT ( 'NONE',  ( 0.9046671180729951578, -5.711843387010016926, 6.579999999999999183 ) ) ;
#6657=CARTESIAN_POINT ( 'NONE',  ( 2.708615832122949652, 5.110351332421781301, 10.06394828327797519 ) ) ;
#6671=CARTESIAN_POINT ( 'NONE',  ( -1.963858260114716980, 4.049832306626327316, 4.043948283277976508 ) ) ;
#6675=CARTESIAN_POINT ( 'NONE',  ( -5.432285873273256627, -0.8603895577212797852, 4.479999999999999538 ) ) ;
#6677=CARTESIAN_POINT ( 'NONE',  ( -0.9046671180729962680, 5.711843387010016926, 10.77999999999999936 ) ) ;
#6683=CARTESIAN_POINT ( 'NONE',  ( -0.8323763977770610722, 4.658724279160015413, 3.376051716722022977 ) ) ;
#6688=CARTESIAN_POINT ( 'NONE',  ( 4.658724279160018966, -0.8323763977770426425, 5.023948283277976046 ) ) ;
#6691=CARTESIAN_POINT ( 'NONE',  ( 5.110351332421769754, 2.708615832122969191, 3.936051716722023031 ) ) ;
#6698=CARTESIAN_POINT ( 'NONE',  ( -4.009529358847660596, 2.042957248827953265, 7.559999999999998721 ) ) ;
#6699=CARTESIAN_POINT ( 'NONE',  ( 4.049832306626335310, -1.963858260114701215, 12.75605171672202331 ) ) ;
#6707=CARTESIAN_POINT ( 'NONE',  ( 2.542276634908080535, 5.195105386651229118, 3.656051716722022782 ) ) ;
#6708=CARTESIAN_POINT ( 'NONE',  ( -0.9046671180729963790, 5.711843387010016926, 2.379999999999999893 ) ) ;
#6709=CARTESIAN_POINT ( 'NONE',  ( -2.496947748567517333, 4.900535883036019058, 10.63999999999999879 ) ) ;
#6717=CARTESIAN_POINT ( 'NONE',  ( -2.231261971483764484, -4.173491630687871101, 11.46394828327797555 ) ) ;
#6720=CARTESIAN_POINT ( 'NONE',  ( -0.8603895577212598011, -5.432285873273260179, 9.519999999999999574 ) ) ;
#6722=CARTESIAN_POINT ( 'NONE',  ( -5.432285873273256627, -0.8603895577212797852, 10.07999999999999829 ) ) ;
#6727=CARTESIAN_POINT ( 'NONE',  ( -0.8323763977770610722, 4.658724279160015413, 8.976051716722020402 ) ) ;
#6730=CARTESIAN_POINT ( 'NONE',  ( 2.708615832122949652, 5.110351332421781301, 1.663948283277976392 ) ) ;
#6735=CARTESIAN_POINT ( 'NONE',  ( -5.110351332421769754, -2.708615832122969191, 8.136051716722024096 ) ) ;
#6736=ADVANCED_BREP_SHAPE_REPRESENTATION ( '', ( #8241, #2101 ), #9398 ) ;
#6742=CARTESIAN_POINT ( 'NONE',  ( -4.673326407553653361, 0.7401821875142517992, 10.21999999999999886 ) ) ;
#6745=CARTESIAN_POINT ( 'NONE',  ( -4.687928535947287756, 0.6479879772514611780, 8.416051716722021681 ) ) ;
#6757=CARTESIAN_POINT ( 'NONE',  ( 2.576046737280769605, -4.860232935257343456, 4.636051716722022320 ) ) ;
#6758=CARTESIAN_POINT ( 'NONE',  ( 4.900535883036028828, -2.496947748567499126, 0.5599999999999999423 ) ) ;
#6759=CARTESIAN_POINT ( 'NONE',  ( -5.711843387010018702, 0.9046671180729746187, 13.01999999999999424 ) ) ;
#6773=CARTESIAN_POINT ( 'NONE',  ( -3.279728542977953687, 3.411736077305369541, 12.30394828327797718 ) ) ;
#6779=CARTESIAN_POINT ( 'NONE',  ( 2.625446233515515537, 5.152728359536502545, 13.85999999999999766 ) ) ;
#6783=CARTESIAN_POINT ( 'NONE',  ( 3.889087296526005488, 3.889087296526018811, 5.599999999999998757 ) ) ;
#6789=CARTESIAN_POINT ( 'NONE',  ( -0.8323763977770610722, 4.658724279160015413, 11.77605171672202289 ) ) ;
#6792=CARTESIAN_POINT ( 'NONE',  ( -0.8124729078102072011, 5.726445515403652209, 1.383948283277976365 ) ) ;
#6795=CARTESIAN_POINT ( 'NONE',  ( 5.110351332421769754, 2.708615832122969191, 1.136051716722023208 ) ) ;
#6799=CARTESIAN_POINT ( 'NONE',  ( 4.444597532678119300, 0.7039550926810472786, 8.679999999999997939 ) ) ;
#6803=CARTESIAN_POINT ( 'NONE',  ( -4.009529358847660596, 2.042957248827953265, 4.759999999999999787 ) ) ;
#6811=CARTESIAN_POINT ( 'NONE',  ( -3.889087296526005044, -3.889087296526019255, 12.59999999999999787 ) ) ;
#6812=CARTESIAN_POINT ( 'NONE',  ( 3.889087296526005488, 3.889087296526018811, 11.19999999999999751 ) ) ;
#6813=CARTESIAN_POINT ( 'NONE',  ( 0.8603895577212593571, 5.432285873273261068, 13.71999999999999886 ) ) ;
#6826=CARTESIAN_POINT ( 'NONE',  ( 4.860232935257354114, -2.576046737280751842, -0.4360517167220233636 ) ) ;
#6831=CARTESIAN_POINT ( 'NONE',  ( -4.089228379062038066, 4.089228379062021190, 10.50000000000000000 ) ) ;
#6838=CARTESIAN_POINT ( 'NONE',  ( 0.8323763977770604061, -4.658724279160015413, 10.37605171672202253 ) ) ;
#6841=CARTESIAN_POINT ( 'NONE',  ( 0.6479879772514793856, -4.687928535947285091, 11.18394828327797441 ) ) ;
#6852=CARTESIAN_POINT ( 'NONE',  ( -2.148092372876330813, -4.215868657802594122, 12.45999999999999730 ) ) ;
#6854=CARTESIAN_POINT ( 'NONE',  ( -2.042957248827969252, 4.009529358847651714, 5.039999999999999147 ) ) ;
#6866=CARTESIAN_POINT ( 'NONE',  ( -4.089228379062038066, 4.089228379062021190, 10.50000000000000000 ) ) ;
#6867=CARTESIAN_POINT ( 'NONE',  ( 5.152728359536493663, 2.625446233515533745, 11.33999999999999808 ) ) ;
#6868=CARTESIAN_POINT ( 'NONE',  ( 4.900535883036028828, -2.496947748567499126, 6.159999999999999254 ) ) ;
#6871=ORIENTED_EDGE ( 'NONE', *, *, #1169, .F. ) ;
#6875=DIRECTION ( 'NONE',  ( -0.7043149233066460235, 0.7043149233066439141, -0.08877487040322810941 ) ) ;
#6881=CARTESIAN_POINT ( 'NONE',  ( 3.279728542977952799, -3.411736077305369541, 5.303948283277975406 ) ) ;
#6885=CARTESIAN_POINT ( 'NONE',  ( -4.089228379062038066, 4.089228379062021190, 13.29999999999999538 ) ) ;
#6892=CARTESIAN_POINT ( 'NONE',  ( -3.411736077305382420, 3.279728542977939476, 11.49605171672201998 ) ) ;
#6894=CARTESIAN_POINT ( 'NONE',  ( 0.8124729078102063129, -5.726445515403652209, 2.783948283277976277 ) ) ;
#6903=CARTESIAN_POINT ( 'NONE',  ( -3.345732310141667831, 3.345732310141653620, 13.29999999999999716 ) ) ;
#6905=CARTESIAN_POINT ( 'NONE',  ( -2.148092372876330813, -4.215868657802593233, 6.859999999999999432 ) ) ;
#6913=CARTESIAN_POINT ( 'NONE',  ( -5.110351332421769754, -2.708615832122969191, 8.136051716722024096 ) ) ;
#6914=CARTESIAN_POINT ( 'NONE',  ( -4.900535883036028828, 2.496947748567499126, 10.35999999999999943 ) ) ;
#6923=DIRECTION ( 'NONE',  ( 0.7071067811865467956, 0.7071067811865484609, 0.000000000000000000 ) ) ;
#6927=CARTESIAN_POINT ( 'NONE',  ( -3.244753828200538148, -3.119207202478392116, 6.003948283277975584 ) ) ;
#6944=CARTESIAN_POINT ( 'NONE',  ( -2.122056237541221968, 3.969226411068977889, 14.43605171672202125 ) ) ;
#6949=CARTESIAN_POINT ( 'NONE',  ( -5.195105386651219348, -2.542276634908102295, 3.343948283277975886 ) ) ;
#6961=CARTESIAN_POINT ( 'NONE',  ( 0.6162731882459174804, 4.458484982038668498, 14.71605171672202239 ) ) ;
#6968=CARTESIAN_POINT ( 'NONE',  ( 5.110351332421769754, 2.708615832122969191, 6.736051716722023741 ) ) ;
#6983=CARTESIAN_POINT ( 'NONE',  ( 4.860232935257354114, -2.576046737280751842, 7.963948283277976437 ) ) ;
#6995=CARTESIAN_POINT ( 'NONE',  ( 2.042957248827968808, -4.009529358847652603, 9.240000000000000213 ) ) ;
#6997=CARTESIAN_POINT ( 'NONE',  ( -5.697241258616385196, 0.9968613283357647958, 12.02394828327797427 ) ) ;
#7010=CARTESIAN_POINT ( 'NONE',  ( 4.009529358847659708, -2.042957248827953709, 11.75999999999999979 ) ) ;
#7019=CARTESIAN_POINT ( 'NONE',  ( 4.155232146225751322, -4.023224611898307934, 7.296051716722023350 ) ) ;
#7036=CARTESIAN_POINT ( 'NONE',  ( 0.9480714621563713917, 5.418398423912717199, 4.323948283277975868 ) ) ;
#7047=CARTESIAN_POINT ( 'NONE',  ( -4.009529358847660596, 2.042957248827953265, 10.35999999999999943 ) ) ;
#7049=CARTESIAN_POINT ( 'NONE',  ( 4.023224611898322145, -4.155232146225737111, 5.303948283277975406 ) ) ;
#7062=CARTESIAN_POINT ( 'NONE',  ( 4.009529358847659708, -2.042957248827953709, 8.959999999999999076 ) ) ;
#7071=CARTESIAN_POINT ( 'NONE',  ( -3.826313983664925811, -3.951860609387098489, 7.996051716722022640 ) ) ;
#7076=CARTESIAN_POINT ( 'NONE',  ( 5.418398423912711870, 0.9480714621563913758, 9.676051716722021467 ) ) ;
#7086=CARTESIAN_POINT ( 'NONE',  ( 0.8124729078102063129, -5.726445515403652209, 2.783948283277976277 ) ) ;
#7090=CARTESIAN_POINT ( 'NONE',  ( 0.000000000000000000, 0.000000000000000000, 0.000000000000000000 ) ) ;
#7100=CARTESIAN_POINT ( 'NONE',  ( -3.345732310141667831, 3.345732310141653620, 4.900000000000000355 ) ) ;
#7103=CARTESIAN_POINT ( 'NONE',  ( 3.951860609387084722, 3.826313983664940022, 4.603948283277976117 ) ) ;
#7118=CARTESIAN_POINT ( 'NONE',  ( 3.181980515339458471, 3.181980515339470461, 13.99999999999999822 ) ) ;
#7127=CARTESIAN_POINT ( 'NONE',  ( 3.826313983664925811, 3.951860609387098044, 12.19605171672202282 ) ) ;
#7133=CARTESIAN_POINT ( 'NONE',  ( 4.049832306626335310, -1.963858260114701215, 1.556051716722023581 ) ) ;
#7141=CARTESIAN_POINT ( 'NONE',  ( -5.446173322633801384, -0.7727076532861678615, 6.283948283277974944 ) ) ;
#7155=CARTESIAN_POINT ( 'NONE',  ( -2.042957248827969252, 4.009529358847651714, 7.839999999999999858 ) ) ;
#7157=CARTESIAN_POINT ( 'NONE',  ( 2.708615832122949652, 5.110351332421781301, 7.263948283277976259 ) ) ;
#7162=CARTESIAN_POINT ( 'NONE',  ( -5.152728359536494551, -2.625446233515535521, 1.540000000000000036 ) ) ;
#7172=CARTESIAN_POINT ( 'NONE',  ( -0.7401821875142701179, 4.673326407553649808, 13.57999999999999474 ) ) ;
#7187=CARTESIAN_POINT ( 'NONE',  ( -4.049832306626335310, 1.963858260114700327, 2.956051716722023492 ) ) ;
#7196=CARTESIAN_POINT ( 'NONE',  ( 4.900535883036028828, -2.496947748567499126, 0.5599999999999999423 ) ) ;
#7198=CARTESIAN_POINT ( 'NONE',  ( -0.9480714621563718358, -5.418398423912716311, 2.923948283277976401 ) ) ;
#7215=CARTESIAN_POINT ( 'NONE',  ( 4.215868657802586128, 2.148092372876346801, 5.739999999999997549 ) ) ;
#7218=CARTESIAN_POINT ( 'NONE',  ( 0.8124729078102063129, -5.726445515403652209, 8.383948283277975477 ) ) ;
#7229=DIRECTION ( 'NONE',  ( 0.7071067811865467956, 0.7071067811865484609, -6.099057733344262077E-17 ) ) ;
#7231=CARTESIAN_POINT ( 'NONE',  ( 0.6479879772514793856, -4.687928535947285091, -0.01605171672202330979 ) ) ;
#7239=CARTESIAN_POINT ( 'NONE',  ( 0.7039550926810297371, 4.444597532678122853, 2.519999999999999574 ) ) ;
#7242=CARTESIAN_POINT ( 'NONE',  ( -0.7727076532861475444, -5.446173322633804048, 13.31605171672202204 ) ) ;
#7249=CARTESIAN_POINT ( 'NONE',  ( -0.8603895577212598011, -5.432285873273260179, 1.119999999999999885 ) ) ;
#7251=CARTESIAN_POINT ( 'NONE',  ( -0.9046671180729963790, 5.711843387010016926, 2.379999999999999893 ) ) ;
#7261=CARTESIAN_POINT ( 'NONE',  ( -4.444597532678119300, -0.7039550926810477227, 12.87999999999999901 ) ) ;
#7267=CARTESIAN_POINT ( 'NONE',  ( 0.9046671180729951578, -5.711843387010016926, 6.579999999999999183 ) ) ;
#7271=CARTESIAN_POINT ( 'NONE',  ( 3.889087296526005488, 3.889087296526018811, 2.799999999999999378 ) ) ;
#7281=CARTESIAN_POINT ( 'NONE',  ( 2.231261971483764484, 4.173491630687871101, 4.463948283277976437 ) ) ;
#7293=CARTESIAN_POINT ( 'NONE',  ( 2.042957248827968808, -4.009529358847652603, 3.639999999999999680 ) ) ;
#7296=CARTESIAN_POINT ( 'NONE',  ( 0.7727076532861471003, 5.446173322633805824, 14.71605171672202239 ) ) ;
#7307=CARTESIAN_POINT ( 'NONE',  ( 5.152728359536493663, 2.625446233515533745, 8.539999999999999147 ) ) ;
#7309=CARTESIAN_POINT ( 'NONE',  ( -2.417848759854264618, 4.940838830814694660, 12.44394828327797597 ) ) ;
#7320=DIRECTION ( 'NONE',  ( -0.7071067811865465735, -0.7071067811865483499, 0.000000000000000000 ) ) ;
#7321=CARTESIAN_POINT ( 'NONE',  ( 4.658724279160018966, -0.8323763977770426425, 2.223948283277975779 ) ) ;
#7324=CARTESIAN_POINT ( 'NONE',  ( -4.900535883036028828, 2.496947748567499126, 4.759999999999999787 ) ) ;
#7331=PRODUCT ( 'spring', 'spring', '', ( #1443 ) ) ;
#7333=CARTESIAN_POINT ( 'NONE',  ( -2.064922774268895811, -4.258245684917318918, 7.856051716722022071 ) ) ;
#7336=CARTESIAN_POINT ( 'NONE',  ( 3.244753828200538148, 3.119207202478391672, 7.403948283277976827 ) ) ;
#7350=CARTESIAN_POINT ( 'NONE',  ( 4.173491630687861331, 2.231261971483781359, 6.736051716722023741 ) ) ;
#7359=CARTESIAN_POINT ( 'NONE',  ( 4.089228379062037178, -4.089228379062022967, 3.499999999999998668 ) ) ;
#7360=CARTESIAN_POINT ( 'NONE',  ( -0.9046671180729963790, 5.711843387010016926, 5.179999999999999716 ) ) ;
#7362=CARTESIAN_POINT ( 'NONE',  ( 0.8603895577212593571, 5.432285873273261068, 2.519999999999999574 ) ) ;
#7373=CARTESIAN_POINT ( 'NONE',  ( -4.009529358847660596, 2.042957248827953265, 13.15999999999999837 ) ) ;
#7376=CARTESIAN_POINT ( 'NONE',  ( 4.900535883036028828, -2.496947748567499126, 8.959999999999999076 ) ) ;
#7379=CARTESIAN_POINT ( 'NONE',  ( 0.8603895577212593571, 5.432285873273261068, 10.91999999999999993 ) ) ;
#7385=CARTESIAN_POINT ( 'NONE',  ( 3.411736077305382420, -3.279728542977940364, 4.496051716722022640 ) ) ;
#7390=CARTESIAN_POINT ( 'NONE',  ( -2.231261971483764484, -4.173491630687871101, 3.063948283277976081 ) ) ;
#7397=CARTESIAN_POINT ( 'NONE',  ( 3.181980515339458471, 3.181980515339470461, 5.599999999999998757 ) ) ;
#7402=CARTESIAN_POINT ( 'NONE',  ( -0.6162731882459178134, -4.458484982038665834, 7.716051716722023279 ) ) ;
#7408=CARTESIAN_POINT ( 'NONE',  ( 2.625446233515515537, 5.152728359536502545, 5.459999999999997300 ) ) ;
#7409=CARTESIAN_POINT ( 'NONE',  ( 0.8603895577212593571, 5.432285873273261068, 5.319999999999999396 ) ) ;
#7410=CARTESIAN_POINT ( 'NONE',  ( -2.708615832122950096, -5.110351332421780413, 11.46394828327797555 ) ) ;
#7418=ORIENTED_EDGE ( 'NONE', *, *, #7662, .T. ) ;
#7421=CARTESIAN_POINT ( 'NONE',  ( 2.042957248827968808, -4.009529358847652603, 12.03999999999999915 ) ) ;
#7424=CARTESIAN_POINT ( 'NONE',  ( 4.900535883036028828, -2.496947748567499126, 0.5599999999999999423 ) ) ;
#7427=CARTESIAN_POINT ( 'NONE',  ( -4.900535883036028828, 2.496947748567499126, 4.759999999999999787 ) ) ;
#7434=CARTESIAN_POINT ( 'NONE',  ( 4.430710083317573655, 0.7916369971161595354, 4.076051716722022711 ) ) ;
#7436=CARTESIAN_POINT ( 'NONE',  ( -0.7916369971161423269, -4.430710083317576320, 8.523948283277976046 ) ) ;
#7443=CARTESIAN_POINT ( 'NONE',  ( -0.9046671180729963790, 5.711843387010016926, 13.57999999999999474 ) ) ;
#7450=CARTESIAN_POINT ( 'NONE',  ( 4.444597532678119300, 0.7039550926810472786, 0.2799999999999999711 ) ) ;
#7454=CARTESIAN_POINT ( 'NONE',  ( -2.122056237541221968, 3.969226411068977889, 6.036051716722022675 ) ) ;
#7465=CARTESIAN_POINT ( 'NONE',  ( -5.432285873273256627, -0.8603895577212797852, 10.07999999999999829 ) ) ;
#7466=CARTESIAN_POINT ( 'NONE',  ( -5.432285873273256627, -0.8603895577212797852, 4.479999999999999538 ) ) ;
#7468=CARTESIAN_POINT ( 'NONE',  ( 4.900535883036028828, -2.496947748567499126, 0.5599999999999999423 ) ) ;
#7483=CARTESIAN_POINT ( 'NONE',  ( 3.244753828200538148, 3.119207202478391672, 1.803948283277976516 ) ) ;
#7486=CARTESIAN_POINT ( 'NONE',  ( 4.089228379062037178, -4.089228379062022967, 3.499999999999998668 ) ) ;
#7489=CARTESIAN_POINT ( 'NONE',  ( -5.432285873273256627, -0.8603895577212797852, 4.479999999999999538 ) ) ;
#7493=CARTESIAN_POINT ( 'NONE',  ( 3.411736077305382420, -3.279728542977940364, 7.296051716722023350 ) ) ;
#7495=CARTESIAN_POINT ( 'NONE',  ( -0.6479879772514802738, 4.687928535947285091, 6.983948283277976010 ) ) ;
#7498=CARTESIAN_POINT ( 'NONE',  ( 0.7727076532861471003, 5.446173322633805824, 3.516051716722023102 ) ) ;
#7503=CARTESIAN_POINT ( 'NONE',  ( 3.181980515339458471, 3.181980515339470461, 11.19999999999999751 ) ) ;
#7507=CARTESIAN_POINT ( 'NONE',  ( -4.430710083317573655, -0.7916369971161599794, 8.276051716722021112 ) ) ;
#7516=CARTESIAN_POINT ( 'NONE',  ( 5.418398423912711870, 0.9480714621563913758, 1.276051716722023333 ) ) ;
#7517=CARTESIAN_POINT ( 'NONE',  ( -4.089228379062038066, 4.089228379062021190, 2.099999999999999201 ) ) ;
#7518=CARTESIAN_POINT ( 'NONE',  ( 3.889087296526005488, 3.889087296526018811, 8.400000000000000355 ) ) ;
#7528=CARTESIAN_POINT ( 'NONE',  ( -4.658724279160018078, 0.8323763977770419764, 9.223948283277977112 ) ) ;
#7536=CARTESIAN_POINT ( 'NONE',  ( -5.152728359536494551, -2.625446233515535521, 9.939999999999997726 ) ) ;
#7542=CARTESIAN_POINT ( 'NONE',  ( 0.8323763977770604061, -4.658724279160015413, 7.576051716722023599 ) ) ;
#7546=CARTESIAN_POINT ( 'NONE',  ( -3.951860609387083834, -3.826313983664940466, 0.4039482832779765498 ) ) ;
#7550=CARTESIAN_POINT ( 'NONE',  ( 0.9968613283357860011, -5.697241258616382531, 7.576051716722023599 ) ) ;
#7556=CARTESIAN_POINT ( 'NONE',  ( 3.181980515339458471, 3.181980515339470461, 8.400000000000000355 ) ) ;
#7557=CARTESIAN_POINT ( 'NONE',  ( -2.122056237541221968, 3.969226411068977889, 8.836051716722023386 ) ) ;
#7561=ORIENTED_EDGE ( 'NONE', *, *, #9280, .T. ) ;
#7565=CARTESIAN_POINT ( 'NONE',  ( 4.940838830814703542, -2.417848759854246410, 4.356051716722023848 ) ) ;
#7566=CARTESIAN_POINT ( 'NONE',  ( 5.152728359536493663, 2.625446233515533745, 0.1399999999999999856 ) ) ;
#7567=CARTESIAN_POINT ( 'NONE',  ( 0.8603895577212593571, 5.432285873273261068, 10.91999999999999993 ) ) ;
#7578=CARTESIAN_POINT ( 'NONE',  ( 2.231261971483764484, 4.173491630687871101, 12.86394828327797768 ) ) ;
#7581=CARTESIAN_POINT ( 'NONE',  ( -0.9046671180729963790, 5.711843387010016926, 10.77999999999999936 ) ) ;
#7583=CARTESIAN_POINT ( 'NONE',  ( 0.9046671180729953798, -5.711843387010016926, 6.579999999999999183 ) ) ;
#7589=CARTESIAN_POINT ( 'NONE',  ( 4.687928535947288644, -0.6479879772514620662, 9.816051716722022036 ) ) ;
#7592=CARTESIAN_POINT ( 'NONE',  ( 4.860232935257354114, -2.576046737280751842, -0.4360517167220233636 ) ) ;
#7595=CARTESIAN_POINT ( 'NONE',  ( 5.726445515403654873, -0.8124729078101852187, 7.016051716722022213 ) ) ;
#7601=CARTESIAN_POINT ( 'NONE',  ( 3.345732310141667387, -3.345732310141654064, 6.299999999999998934 ) ) ;
#7604=CARTESIAN_POINT ( 'NONE',  ( 0.7039550926810297371, 4.444597532678122853, 2.519999999999999574 ) ) ;
#7608=SHAPE_REPRESENTATION ( 'spring', ( #2101 ), #9398 ) ;
#7617=CARTESIAN_POINT ( 'NONE',  ( 4.940838830814703542, -2.417848759854246410, 1.556051716722023581 ) ) ;
#7618=CARTESIAN_POINT ( 'NONE',  ( 0.9046671180729951578, -5.711843387010016926, 12.17999999999999439 ) ) ;
#7619=CARTESIAN_POINT ( 'NONE',  ( -2.496947748567517333, 4.900535883036019058, 13.43999999999999950 ) ) ;
#7635=CARTESIAN_POINT ( 'NONE',  ( 4.258245684917310037, 2.064922774268912686, 10.34394828327797633 ) ) ;
#7639=CARTESIAN_POINT ( 'NONE',  ( 0.8603895577212593571, 5.432285873273261068, 13.71999999999999886 ) ) ;
#7644=CARTESIAN_POINT ( 'NONE',  ( -5.152728359536494551, -2.625446233515535521, 12.73999999999999844 ) ) ;
#7648=CARTESIAN_POINT ( 'NONE',  ( -3.119207202478379681, -3.244753828200550139, 10.79605171672202246 ) ) ;
#7650=CARTESIAN_POINT ( 'NONE',  ( -2.708615832122950096, -5.110351332421780413, 0.2639482832779765920 ) ) ;
#7657=CARTESIAN_POINT ( 'NONE',  ( 2.148092372876330369, 4.215868657802594122, 11.05999999999999872 ) ) ;
#7659=CARTESIAN_POINT ( 'NONE',  ( 3.345732310141667387, -3.345732310141653620, 3.499999999999998668 ) ) ;
#7662=EDGE_CURVE ( 'NONE', #5138, #8250, #1179, .T. ) ;
#7672=CARTESIAN_POINT ( 'NONE',  ( 2.576046737280769605, -4.860232935257343456, 1.836051716722023386 ) ) ;
#7673=CARTESIAN_POINT ( 'NONE',  ( -4.900535883036028828, 2.496947748567499126, 13.15999999999999837 ) ) ;
#7674=CARTESIAN_POINT ( 'NONE',  ( 0.8603895577212593571, 5.432285873273261068, 5.319999999999999396 ) ) ;
#7689=CARTESIAN_POINT ( 'NONE',  ( -1.963858260114716980, 4.049832306626327316, 9.643948283277975264 ) ) ;
#7701=CARTESIAN_POINT ( 'NONE',  ( 3.181980515339458471, 3.181980515339470461, 2.232096619617652273E-17 ) ) ;
#7703=CARTESIAN_POINT ( 'NONE',  ( 2.231261971483764484, 4.173491630687871101, 10.06394828327797519 ) ) ;
#7713=CIRCLE ( 'NONE', #1110, 0.5000000000000000000 ) ;
#7715=CARTESIAN_POINT ( 'NONE',  ( -4.673326407553653361, 0.7401821875142517992, 13.01999999999999602 ) ) ;
#7716=CARTESIAN_POINT ( 'NONE',  ( 0.7401821875142697849, -4.673326407553650697, 6.579999999999999183 ) ) ;
#7727=CARTESIAN_POINT ( 'NONE',  ( -2.576046737280769605, 4.860232935257343456, 8.836051716722023386 ) ) ;
#7729=CARTESIAN_POINT ( 'NONE',  ( 2.496947748567516889, -4.900535883036019946, 9.240000000000000213 ) ) ;
#7730=CARTESIAN_POINT ( 'NONE',  ( -0.8603895577212598011, -5.432285873273260179, 6.719999999999999751 ) ) ;
#7740=CARTESIAN_POINT ( 'NONE',  ( 2.231261971483764484, 4.173491630687871101, 10.06394828327797519 ) ) ;
#7752=CARTESIAN_POINT ( 'NONE',  ( -4.215868657802586128, -2.148092372876348133, 1.540000000000000036 ) ) ;
#7754=CARTESIAN_POINT ( 'NONE',  ( 2.231261971483764484, 4.173491630687871101, 12.86394828327797768 ) ) ;
#7758=CARTESIAN_POINT ( 'NONE',  ( 3.889087296526005488, 3.889087296526018811, -3.866961113726609188E-17 ) ) ;
#7765=CARTESIAN_POINT ( 'NONE',  ( 2.042957248827968808, -4.009529358847652603, 3.639999999999999680 ) ) ;
#7773=CARTESIAN_POINT ( 'NONE',  ( -5.726445515403654873, 0.8124729078101847746, 5.616051716722022746 ) ) ;
#7788=CARTESIAN_POINT ( 'NONE',  ( -4.860232935257354114, 2.576046737280751842, 3.763948283277976703 ) ) ;
#7790=AXIS2_PLACEMENT_3D ( 'NONE', #420, #6875, #6923 ) ;
#7805=CARTESIAN_POINT ( 'NONE',  ( -0.8323763977770610722, 4.658724279160015413, 14.57605171672202538 ) ) ;
#7809=CARTESIAN_POINT ( 'NONE',  ( -2.417848759854264618, 4.940838830814694660, 6.843948283277976330 ) ) ;
#7822=CARTESIAN_POINT ( 'NONE',  ( -4.049832306626335310, 1.963858260114700327, 14.15605171672202012 ) ) ;
#7829=CARTESIAN_POINT ( 'NONE',  ( 5.418398423912711870, 0.9480714621563913758, 12.47605171672202218 ) ) ;
#7839=CARTESIAN_POINT ( 'NONE',  ( 4.023224611898322145, -4.155232146225737111, 5.303948283277975406 ) ) ;
#7851=CARTESIAN_POINT ( 'NONE',  ( 3.181980515339458471, 3.181980515339470461, 5.599999999999998757 ) ) ;
#7855=CARTESIAN_POINT ( 'NONE',  ( -5.446173322633801384, -0.7727076532861678615, 9.083948283277974767 ) ) ;
#7870=CARTESIAN_POINT ( 'NONE',  ( -4.444597532678119300, -0.7039550926810477227, 7.279999999999999361 ) ) ;
#7872=PRODUCT_DEFINITION_FORMATION_WITH_SPECIFIED_SOURCE ( 'ANY', '', #7331, .NOT_KNOWN. ) ;
#7877=FILL_AREA_STYLE ('',( #9531 ) ) ;
#7879=CARTESIAN_POINT ( 'NONE',  ( -2.542276634908081423, -5.195105386651227342, 13.45605171672202260 ) ) ;
#7884=CARTESIAN_POINT ( 'NONE',  ( -4.155232146225753098, 4.023224611898306158, 11.49605171672201998 ) ) ;
#7895=CARTESIAN_POINT ( 'NONE',  ( -2.417848759854264618, 4.940838830814694660, 6.843948283277976330 ) ) ;
#7907=CARTESIAN_POINT ( 'NONE',  ( 0.7401821875142697849, -4.673326407553650697, 3.779999999999998472 ) ) ;
#7909=CARTESIAN_POINT ( 'NONE',  ( -5.697241258616385196, 0.9968613283357647958, 9.223948283277977112 ) ) ;
#7922=CARTESIAN_POINT ( 'NONE',  ( -3.181980515339458027, -3.181980515339470905, 6.999999999999999112 ) ) ;
#7931=CARTESIAN_POINT ( 'NONE',  ( -3.826313983664925811, -3.951860609387098489, 10.79605171672202246 ) ) ;
#7935=CARTESIAN_POINT ( 'NONE',  ( 3.826313983664925811, 3.951860609387098044, 12.19605171672202282 ) ) ;
#7945=CARTESIAN_POINT ( 'NONE',  ( -3.951860609387083834, -3.826313983664940466, 3.203948283277977094 ) ) ;
#7962=CARTESIAN_POINT ( 'NONE',  ( -4.673326407553653361, 0.7401821875142517992, 7.419999999999998153 ) ) ;
#7965=CARTESIAN_POINT ( 'NONE',  ( 5.446173322633801384, 0.7727076532861675284, 7.683948283277975300 ) ) ;
#7982=CARTESIAN_POINT ( 'NONE',  ( -3.181980515339458027, -3.181980515339470905, 9.799999999999998934 ) ) ;
#7997=CARTESIAN_POINT ( 'NONE',  ( -2.064922774268895811, -4.258245684917318918, 2.256051716722022871 ) ) ;
#8003=CARTESIAN_POINT ( 'NONE',  ( 4.900535883036028828, -2.496947748567499126, 6.159999999999999254 ) ) ;
#8005=CARTESIAN_POINT ( 'NONE',  ( -5.697241258616385196, 0.9968613283357647958, 0.8239482832779764232 ) ) ;
#8018=CARTESIAN_POINT ( 'NONE',  ( 4.673326407553653361, -0.7401821875142523544, 3.219999999999999751 ) ) ;
#8021=CARTESIAN_POINT ( 'NONE',  ( 5.697241258616385196, -0.9968613283357656840, 5.023948283277976046 ) ) ;
#8036=CARTESIAN_POINT ( 'NONE',  ( 3.279728542977952799, -3.411736077305369541, -0.2960517167220233503 ) ) ;
#8049=CARTESIAN_POINT ( 'NONE',  ( 0.6162731882459174804, 4.458484982038668498, 3.516051716722023102 ) ) ;
#8059=CARTESIAN_POINT ( 'NONE',  ( 5.711843387010018702, -0.9046671180729751738, 8.820000000000000284 ) ) ;
#8061=CARTESIAN_POINT ( 'NONE',  ( -4.900535883036028828, 2.496947748567499126, 4.759999999999999787 ) ) ;
#8073=CARTESIAN_POINT ( 'NONE',  ( 4.009529358847659708, -2.042957248827953709, 6.159999999999999254 ) ) ;
#8076=CARTESIAN_POINT ( 'NONE',  ( -5.152728359536494551, -2.625446233515535077, 7.139999999999997016 ) ) ;
#8086=CARTESIAN_POINT ( 'NONE',  ( 4.673326407553653361, -0.7401821875142523544, 11.61999999999999922 ) ) ;
#8096=CARTESIAN_POINT ( 'NONE',  ( 2.148092372876330369, 4.215868657802594122, 2.659999999999999254 ) ) ;
#8099=CARTESIAN_POINT ( 'NONE',  ( 3.826313983664925811, 3.951860609387098044, 9.396051716722022107 ) ) ;
#8107=CARTESIAN_POINT ( 'NONE',  ( -4.900535883036028828, 2.496947748567499126, 7.559999999999998721 ) ) ;
#8109=CARTESIAN_POINT ( 'NONE',  ( 0.9046671180729951578, -5.711843387010016926, 0.9799999999999997602 ) ) ;
#8120=CARTESIAN_POINT ( 'NONE',  ( 3.181980515339458471, 3.181980515339470461, 2.232096619617652273E-17 ) ) ;
#8121=CARTESIAN_POINT ( 'NONE',  ( -2.042957248827969252, 4.009529358847651714, 13.43999999999999950 ) ) ;
#8127=CARTESIAN_POINT ( 'NONE',  ( -0.9046671180729963790, 5.711843387010016926, 5.179999999999999716 ) ) ;
#8138=CARTESIAN_POINT ( 'NONE',  ( -4.049832306626335310, 1.963858260114700327, 2.956051716722023492 ) ) ;
#8142=CARTESIAN_POINT ( 'NONE',  ( -3.244753828200538148, -3.119207202478392116, 6.003948283277975584 ) ) ;
#8151=CARTESIAN_POINT ( 'NONE',  ( 3.181980515339458471, 3.181980515339470461, 3.651811961182260059E-17 ) ) ;
#8155=CARTESIAN_POINT ( 'NONE',  ( 0.8323763977770604061, -4.658724279160015413, 7.576051716722023599 ) ) ;
#8164=CARTESIAN_POINT ( 'NONE',  ( 5.152728359536493663, 2.625446233515533745, 2.939999999999999059 ) ) ;
#8166=CARTESIAN_POINT ( 'NONE',  ( -4.023224611898323033, 4.155232146225737111, 12.30394828327797718 ) ) ;
#8176=CARTESIAN_POINT ( 'NONE',  ( -3.969226411068985882, 2.122056237541205537, 3.763948283277976703 ) ) ;
#8179=CARTESIAN_POINT ( 'NONE',  ( -2.625446233515515981, -5.152728359536500768, 6.859999999999999432 ) ) ;
#8182=CARTESIAN_POINT ( 'NONE',  ( 4.900535883036028828, -2.496947748567499126, 8.959999999999999076 ) ) ;
#8190=CARTESIAN_POINT ( 'NONE',  ( 3.119207202478379681, 3.244753828200549695, 0.9960517167220231949 ) ) ;
#8191=CARTESIAN_POINT ( 'NONE',  ( 3.535533905932731980, 3.535533905932744414, -8.174322470544786116E-18 ) ) ;
#8192=CARTESIAN_POINT ( 'NONE',  ( -3.244753828200538148, -3.119207202478392116, 8.803948283277977183 ) ) ;
#8205=CARTESIAN_POINT ( 'NONE',  ( -0.6162731882459178134, -4.458484982038665834, 4.916051716722023457 ) ) ;
#8213=CARTESIAN_POINT ( 'NONE',  ( -5.432285873273256627, -0.8603895577212797852, 1.679999999999999938 ) ) ;
#8214=CARTESIAN_POINT ( 'NONE',  ( 4.900535883036028828, -2.496947748567499126, 3.359999999999999876 ) ) ;
#8216=CARTESIAN_POINT ( 'NONE',  ( -5.446173322633801384, -0.7727076532861678615, 11.88394828327797548 ) ) ;
#8230=CARTESIAN_POINT ( 'NONE',  ( 2.231261971483764484, 4.173491630687871101, 1.663948283277976392 ) ) ;
#8233=CARTESIAN_POINT ( 'NONE',  ( -3.889087296526005044, -3.889087296526019255, 4.200000000000000178 ) ) ;
#8238=CARTESIAN_POINT ( 'NONE',  ( 4.089228379062037178, -4.089228379062022967, 9.099999999999996092 ) ) ;
#8241=MANIFOLD_SOLID_BREP ( 'Sweep1', #4551 ) ;
#8244=CARTESIAN_POINT ( 'NONE',  ( 2.064922774268895811, 4.258245684917319807, 3.656051716722022782 ) ) ;
#8246=CARTESIAN_POINT ( 'NONE',  ( -3.279728542977953687, 3.411736077305369541, 9.503948283277974696 ) ) ;
#8250=VERTEX_POINT ( 'NONE', #4008 ) ;
#8251=CARTESIAN_POINT ( 'NONE',  ( 4.940838830814703542, -2.417848759854246410, 1.556051716722023581 ) ) ;
#8257=CARTESIAN_POINT ( 'NONE',  ( -2.122056237541221968, 3.969226411068977889, 11.63605171672202232 ) ) ;
#8267=CARTESIAN_POINT ( 'NONE',  ( -5.110351332421769754, -2.708615832122969191, 2.536051716722023119 ) ) ;
#8268=CARTESIAN_POINT ( 'NONE',  ( -5.152728359536494551, -2.625446233515535077, 1.540000000000000036 ) ) ;
#8269=CARTESIAN_POINT ( 'NONE',  ( -0.8603895577212598011, -5.432285873273260179, 3.919999999999999929 ) ) ;
#8281=CARTESIAN_POINT ( 'NONE',  ( 3.969226411068985882, -2.122056237541205981, -0.4360517167220233636 ) ) ;
#8285=CARTESIAN_POINT ( 'NONE',  ( -4.089228379062038066, 4.089228379062021190, 4.900000000000000355 ) ) ;
#8287=CARTESIAN_POINT ( 'NONE',  ( 2.496947748567516889, -4.900535883036019946, 9.240000000000000213 ) ) ;
#8292=CARTESIAN_POINT ( 'NONE',  ( -5.726445515403654873, 0.8124729078101847746, 14.01605171672202310 ) ) ;
#8295=CARTESIAN_POINT ( 'NONE',  ( -0.7916369971161423269, -4.430710083317576320, 5.723948283277976223 ) ) ;
#8299=CARTESIAN_POINT ( 'NONE',  ( -5.726445515403654873, 0.8124729078101847746, 5.616051716722022746 ) ) ;
#8309=CARTESIAN_POINT ( 'NONE',  ( 2.122056237541221524, -3.969226411068978777, 13.03605171672202090 ) ) ;
#8320=CARTESIAN_POINT ( 'NONE',  ( 4.155232146225751322, -4.023224611898307934, 1.696051716722023484 ) ) ;
#8322=CARTESIAN_POINT ( 'NONE',  ( 0.8603895577212593571, 5.432285873273261068, 8.119999999999999218 ) ) ;
#8324=CARTESIAN_POINT ( 'NONE',  ( 4.900535883036028828, -2.496947748567499126, 8.959999999999999076 ) ) ;
#8337=CARTESIAN_POINT ( 'NONE',  ( 0.7916369971161419938, 4.430710083317576320, 9.923948283277976401 ) ) ;
#8342=CARTESIAN_POINT ( 'NONE',  ( -0.9046671180729962680, 5.711843387010016926, 5.179999999999999716 ) ) ;
#8346=CARTESIAN_POINT ( 'NONE',  ( -3.119207202478379681, -3.244753828200550139, 7.996051716722022640 ) ) ;
#8349=CARTESIAN_POINT ( 'NONE',  ( 3.969226411068985882, -2.122056237541205981, 2.363948283277975904 ) ) ;
#8352=CARTESIAN_POINT ( 'NONE',  ( -5.726445515403654873, 0.8124729078101847746, 2.816051716722022924 ) ) ;
#8359=CARTESIAN_POINT ( 'NONE',  ( 2.064922774268895811, 4.258245684917319807, 6.456051716722022604 ) ) ;
#8368=CARTESIAN_POINT ( 'NONE',  ( -5.152728359536494551, -2.625446233515535077, 9.939999999999994174 ) ) ;
#8370=CARTESIAN_POINT ( 'NONE',  ( 0.8603895577212593571, 5.432285873273261068, 8.119999999999999218 ) ) ;
#8383=CARTESIAN_POINT ( 'NONE',  ( -1.963858260114716980, 4.049832306626327316, 6.843948283277976330 ) ) ;
#8387=CARTESIAN_POINT ( 'NONE',  ( -2.625446233515515981, -5.152728359536500768, 9.659999999999994813 ) ) ;
#8391=CARTESIAN_POINT ( 'NONE',  ( -4.900535883036028828, 2.496947748567499126, 10.35999999999999943 ) ) ;
#8396=CARTESIAN_POINT ( 'NONE',  ( 2.122056237541221524, -3.969226411068978777, 10.23605171672202374 ) ) ;
#8399=CARTESIAN_POINT ( 'NONE',  ( 3.951860609387084722, 3.826313983664940022, -0.9960517167220231949 ) ) ;
#8404=CARTESIAN_POINT ( 'NONE',  ( -4.940838830814703542, 2.417848759854245078, 5.756051716722022427 ) ) ;
#8410=CARTESIAN_POINT ( 'NONE',  ( 4.444597532678119300, 0.7039550926810472786, 11.47999999999999865 ) ) ;
#8412=CARTESIAN_POINT ( 'NONE',  ( 4.215868657802586128, 2.148092372876346801, 0.1400000000000000411 ) ) ;
#8421=CARTESIAN_POINT ( 'NONE',  ( -5.432285873273256627, -0.8603895577212797852, 12.87999999999999901 ) ) ;
#8422=CARTESIAN_POINT ( 'NONE',  ( -5.711843387010018702, 0.9046671180729746187, 4.620000000000000107 ) ) ;
#8423=CARTESIAN_POINT ( 'NONE',  ( -2.496947748567517333, 4.900535883036019058, 5.039999999999999147 ) ) ;
#8435=CARTESIAN_POINT ( 'NONE',  ( 5.697241258616385196, -0.9968613283357656840, -0.5760517167220230439 ) ) ;
#8438=CARTESIAN_POINT ( 'NONE',  ( 2.625446233515515537, 5.152728359536502545, 11.05999999999999872 ) ) ;
#8444=CARTESIAN_POINT ( 'NONE',  ( 0.6162731882459174804, 4.458484982038668498, 9.116051716722020970 ) ) ;
#8448=CARTESIAN_POINT ( 'NONE',  ( 2.417848759854264618, -4.940838830814695548, -0.1560517167220233370 ) ) ;
#8451=CARTESIAN_POINT ( 'NONE',  ( 0.9968613283357860011, -5.697241258616382531, 4.776051716722021112 ) ) ;
#8456=CARTESIAN_POINT ( 'NONE',  ( -0.7401821875142703400, 4.673326407553649808, 10.77999999999999936 ) ) ;
#8458=CARTESIAN_POINT ( 'NONE',  ( 2.064922774268895811, 4.258245684917319807, 14.85605171672202296 ) ) ;
#8471=CARTESIAN_POINT ( 'NONE',  ( 4.089228379062037178, -4.089228379062022967, 11.90000000000000036 ) ) ;
#8472=CARTESIAN_POINT ( 'NONE',  ( 0.8603895577212593571, 5.432285873273261068, 10.91999999999999993 ) ) ;
#8473=CARTESIAN_POINT ( 'NONE',  ( 2.496947748567516889, -4.900535883036019946, 9.240000000000000213 ) ) ;
#8486=CARTESIAN_POINT ( 'NONE',  ( 3.279728542977952799, -3.411736077305369541, 8.103948283277974340 ) ) ;
#8497=CARTESIAN_POINT ( 'NONE',  ( -3.411736077305382420, 3.279728542977939476, 14.29605171672202424 ) ) ;
#8499=CARTESIAN_POINT ( 'NONE',  ( -5.195105386651219348, -2.542276634908102295, 0.5439482832779766186 ) ) ;
#8509=CARTESIAN_POINT ( 'NONE',  ( -0.7401821875142703400, 4.673326407553649808, 7.979999999999999538 ) ) ;
#8511=CARTESIAN_POINT ( 'NONE',  ( 4.009529358847659708, -2.042957248827953709, 6.159999999999999254 ) ) ;
#8522=CARTESIAN_POINT ( 'NONE',  ( 5.110351332421769754, 2.708615832122969191, 12.33605171672202339 ) ) ;
#8523=CARTESIAN_POINT ( 'NONE',  ( 0.9046671180729951578, -5.711843387010016926, 9.379999999999995453 ) ) ;
#8524=CARTESIAN_POINT ( 'NONE',  ( 2.625446233515515537, 5.152728359536502545, 11.05999999999999872 ) ) ;
#8536=CARTESIAN_POINT ( 'NONE',  ( 4.458484982038663169, 0.6162731882459350219, 7.683948283277975300 ) ) ;
#8547=CARTESIAN_POINT ( 'NONE',  ( -2.148092372876330813, -4.215868657802593233, 1.259999999999999787 ) ) ;
#8551=CARTESIAN_POINT ( 'NONE',  ( 3.969226411068985882, -2.122056237541205981, 10.76394828327797626 ) ) ;
#8563=CARTESIAN_POINT ( 'NONE',  ( 4.009529358847659708, -2.042957248827953709, 3.359999999999999876 ) ) ;
#8568=EDGE_LOOP ( 'NONE', ( #8619, #9479, #7418, #4774 ) ) ;
#8573=CARTESIAN_POINT ( 'NONE',  ( -2.542276634908081423, -5.195105386651227342, 7.856051716722022071 ) ) ;
#8586=CARTESIAN_POINT ( 'NONE',  ( -2.708615832122950096, -5.110351332421780413, 5.863948283277976792 ) ) ;
#8596=CARTESIAN_POINT ( 'NONE',  ( 2.064922774268895811, 4.258245684917319807, 9.256051716722023315 ) ) ;
#8598=CARTESIAN_POINT ( 'NONE',  ( 5.446173322633801384, 0.7727076532861675284, 4.883948283277976365 ) ) ;
#8607=CARTESIAN_POINT ( 'NONE',  ( 3.181980515339458471, 3.181980515339470461, 5.599999999999998757 ) ) ;
#8616=CARTESIAN_POINT ( 'NONE',  ( 2.576046737280769605, -4.860232935257343456, 10.23605171672202374 ) ) ;
#8619=ORIENTED_EDGE ( 'NONE', *, *, #6417, .T. ) ;
#8633=CARTESIAN_POINT ( 'NONE',  ( -2.708615832122950096, -5.110351332421780413, 8.663948283277974838 ) ) ;
#8649=CARTESIAN_POINT ( 'NONE',  ( 2.148092372876330369, 4.215868657802593233, 8.259999999999999787 ) ) ;
#8653=CARTESIAN_POINT ( 'NONE',  ( -2.417848759854264618, 4.940838830814694660, 12.44394828327797597 ) ) ;
#8665=CARTESIAN_POINT ( 'NONE',  ( -2.148092372876330813, -4.215868657802593233, 12.45999999999999552 ) ) ;
#8670=PRESENTATION_STYLE_ASSIGNMENT (( #6275 ) ) ;
#8673=CARTESIAN_POINT ( 'NONE',  ( 2.576046737280769605, -4.860232935257343456, 13.03605171672202090 ) ) ;
#8676=CARTESIAN_POINT ( 'NONE',  ( -4.155232146225753098, 4.023224611898306158, 14.29605171672202424 ) ) ;
#8686=CARTESIAN_POINT ( 'NONE',  ( 2.417848759854264618, -4.940838830814695548, 2.643948283277976596 ) ) ;
#8698=CARTESIAN_POINT ( 'NONE',  ( 2.148092372876330369, 4.215868657802593233, 2.659999999999998366 ) ) ;
#8701=CARTESIAN_POINT ( 'NONE',  ( -3.951860609387083834, -3.826313983664940466, 11.60394828327797434 ) ) ;
#8713=CARTESIAN_POINT ( 'NONE',  ( -4.444597532678119300, -0.7039550926810477227, 12.87999999999999901 ) ) ;
#8722=CARTESIAN_POINT ( 'NONE',  ( 2.576046737280769605, -4.860232935257343456, 7.436051716722023031 ) ) ;
#8728=CARTESIAN_POINT ( 'NONE',  ( 2.542276634908080535, 5.195105386651229118, 14.85605171672202296 ) ) ;
#8740=CARTESIAN_POINT ( 'NONE',  ( 3.951860609387084722, 3.826313983664940022, 1.803948283277976516 ) ) ;
#8752=CARTESIAN_POINT ( 'NONE',  ( -3.181980515339458027, -3.181980515339470905, 4.200000000000000178 ) ) ;
#8754=CARTESIAN_POINT ( 'NONE',  ( 5.152728359536493663, 2.625446233515533745, 0.1399999999999999856 ) ) ;
#8758=CARTESIAN_POINT ( 'NONE',  ( 3.889087296526005488, 3.889087296526018811, -3.866961113726609188E-17 ) ) ;
#8769=CARTESIAN_POINT ( 'NONE',  ( -0.7039550926810301812, -4.444597532678121965, 12.31999999999999851 ) ) ;
#8777=CARTESIAN_POINT ( 'NONE',  ( 2.542276634908080535, 5.195105386651229118, 14.85605171672202296 ) ) ;
#8782=CARTESIAN_POINT ( 'NONE',  ( 2.576046737280769605, -4.860232935257343456, 13.03605171672202090 ) ) ;
#8791=DIRECTION ( 'NONE',  ( -0.7043149233066460235, 0.7043149233066439141, -0.08877487040322810941 ) ) ;
#8793=CARTESIAN_POINT ( 'NONE',  ( -3.951860609387083834, -3.826313983664940466, 0.4039482832779765498 ) ) ;
#8807=CARTESIAN_POINT ( 'NONE',  ( 4.215868657802586128, 2.148092372876346801, 11.33999999999999808 ) ) ;
#8810=CARTESIAN_POINT ( 'NONE',  ( -5.446173322633801384, -0.7727076532861678615, 6.283948283277974944 ) ) ;
#8817=CARTESIAN_POINT ( 'NONE',  ( -2.496947748567517333, 4.900535883036019058, 2.239999999999999769 ) ) ;
#8825=CARTESIAN_POINT ( 'NONE',  ( 3.969226411068985882, -2.122056237541205981, -0.4360517167220233636 ) ) ;
#8840=CARTESIAN_POINT ( 'NONE',  ( 2.122056237541221524, -3.969226411068978777, 1.836051716722023386 ) ) ;
#8848=CARTESIAN_POINT ( 'NONE',  ( 0.8603895577212593571, 5.432285873273261068, 8.119999999999999218 ) ) ;
#8850=CARTESIAN_POINT ( 'NONE',  ( 5.711843387010018702, -0.9046671180729751738, 0.4199999999999999289 ) ) ;
#8861=CARTESIAN_POINT ( 'NONE',  ( 4.444597532678119300, 0.7039550926810472786, 5.879999999999999893 ) ) ;
#8865=CARTESIAN_POINT ( 'NONE',  ( -3.889087296526005044, -3.889087296526019255, 6.999999999999999112 ) ) ;
#8878=CARTESIAN_POINT ( 'NONE',  ( -4.458484982038663169, -0.6162731882459353550, 0.6839482832779766319 ) ) ;
#8891=CARTESIAN_POINT ( 'NONE',  ( 4.430710083317573655, 0.7916369971161595354, 4.076051716722022711 ) ) ;
#8898=CARTESIAN_POINT ( 'NONE',  ( 5.152728359536493663, 2.625446233515533745, 5.739999999999997549 ) ) ;
#8901=CARTESIAN_POINT ( 'NONE',  ( 2.708615832122949652, 5.110351332421781301, 12.86394828327797768 ) ) ;
#8914=CARTESIAN_POINT ( 'NONE',  ( -3.279728542977953687, 3.411736077305369541, 3.903948283277975939 ) ) ;
#8918=CARTESIAN_POINT ( 'NONE',  ( 5.152728359536493663, 2.625446233515533745, 5.739999999999997549 ) ) ;
#8927=CARTESIAN_POINT ( 'NONE',  ( -4.458484982038663169, -0.6162731882459353550, 3.483948283277976898 ) ) ;
#8937=CARTESIAN_POINT ( 'NONE',  ( -4.430710083317573655, -0.7916369971161599794, 11.07605171672202182 ) ) ;
#8946=CARTESIAN_POINT ( 'NONE',  ( 2.496947748567516889, -4.900535883036019946, 3.639999999999999680 ) ) ;
#8948=CARTESIAN_POINT ( 'NONE',  ( 4.089228379062037178, -4.089228379062022967, 0.6999999999999997335 ) ) ;
#8954=AXIS2_PLACEMENT_3D ( 'NONE', #8120, #6515, #7320 ) ;
#8961=CARTESIAN_POINT ( 'NONE',  ( 2.148092372876330369, 4.215868657802593233, 13.85999999999999766 ) ) ;
#8966=CARTESIAN_POINT ( 'NONE',  ( 2.625446233515515537, 5.152728359536502545, 5.459999999999997300 ) ) ;
#8978=CARTESIAN_POINT ( 'NONE',  ( -4.687928535947287756, 0.6479879772514611780, 2.816051716722022924 ) ) ;
#8980=COLOUR_RGB ( '', 0.31764706, 0.68627451, 0.89019608) ;
#8981=CARTESIAN_POINT ( 'NONE',  ( -4.658724279160018078, 0.8323763977770419764, 0.8239482832779764232 ) ) ;
#8991=CARTESIAN_POINT ( 'NONE',  ( 2.148092372876330369, 4.215868657802594122, 5.459999999999999076 ) ) ;
#8995=CARTESIAN_POINT ( 'NONE',  ( 4.687928535947288644, -0.6479879772514620662, 7.016051716722022213 ) ) ;
#9004=CARTESIAN_POINT ( 'NONE',  ( -0.9046671180729963790, 5.711843387010016926, 5.179999999999999716 ) ) ;
#9005=CARTESIAN_POINT ( 'NONE',  ( -4.900535883036028828, 2.496947748567499126, 1.959999999999999964 ) ) ;
#9006=CARTESIAN_POINT ( 'NONE',  ( 5.195105386651219348, 2.542276634908100075, 10.34394828327797633 ) ) ;
#9018=CARTESIAN_POINT ( 'NONE',  ( -2.148092372876330813, -4.215868657802593233, 12.45999999999999552 ) ) ;
#9024=CARTESIAN_POINT ( 'NONE',  ( 5.711843387010018702, -0.9046671180729751738, 3.219999999999999751 ) ) ;
#9026=CARTESIAN_POINT ( 'NONE',  ( 2.625446233515515093, 5.152728359536503433, 11.05999999999999872 ) ) ;
#9032=CARTESIAN_POINT ( 'NONE',  ( 2.064922774268895811, 4.258245684917319807, 6.456051716722022604 ) ) ;
#9035=CARTESIAN_POINT ( 'NONE',  ( -4.658724279160018078, 0.8323763977770419764, 9.223948283277977112 ) ) ;
#9039=CARTESIAN_POINT ( 'NONE',  ( -2.542276634908081423, -5.195105386651227342, 7.856051716722022071 ) ) ;
#9046=CARTESIAN_POINT ( 'NONE',  ( -3.345732310141667831, 3.345732310141653620, 4.899999999999999467 ) ) ;
#9049=CARTESIAN_POINT ( 'NONE',  ( -3.411736077305382420, 3.279728542977939476, 11.49605171672201998 ) ) ;
#9054=CARTESIAN_POINT ( 'NONE',  ( 3.535533905932731980, 3.535533905932744414, -8.174322470544786116E-18 ) ) ;
#9057=CARTESIAN_POINT ( 'NONE',  ( -5.152728359536494551, -2.625446233515535077, 4.339999999999999858 ) ) ;
#9058=CARTESIAN_POINT ( 'NONE',  ( -5.152728359536494551, -2.625446233515535077, 7.139999999999997016 ) ) ;
#9060=CARTESIAN_POINT ( 'NONE',  ( 5.697241258616385196, -0.9968613283357656840, 10.62394828327797569 ) ) ;
#9075=CARTESIAN_POINT ( 'NONE',  ( -4.458484982038663169, -0.6162731882459353550, 0.6839482832779766319 ) ) ;
#9078=CARTESIAN_POINT ( 'NONE',  ( 4.900535883036028828, -2.496947748567499126, 3.359999999999999876 ) ) ;
#9081=CARTESIAN_POINT ( 'NONE',  ( -2.625446233515515537, -5.152728359536502545, 6.859999999999999432 ) ) ;
#9087=CARTESIAN_POINT ( 'NONE',  ( -3.119207202478379681, -3.244753828200550139, 2.396051716722022551 ) ) ;
#9089=CARTESIAN_POINT ( 'NONE',  ( -1.963858260114716980, 4.049832306626327316, 1.243948283277976463 ) ) ;
#9092=CARTESIAN_POINT ( 'NONE',  ( -2.542276634908081423, -5.195105386651227342, 5.056051716722023137 ) ) ;
#9100=CARTESIAN_POINT ( 'NONE',  ( -4.430710083317573655, -0.7916369971161599794, 5.476051716722023066 ) ) ;
#9109=CARTESIAN_POINT ( 'NONE',  ( -2.496947748567517333, 4.900535883036019058, 10.63999999999999879 ) ) ;
#9110=CARTESIAN_POINT ( 'NONE',  ( -4.089228379062038066, 4.089228379062021190, 7.699999999999998401 ) ) ;
#9111=CARTESIAN_POINT ( 'NONE',  ( 5.152728359536493663, 2.625446233515533745, 5.739999999999997549 ) ) ;
#9121=CARTESIAN_POINT ( 'NONE',  ( 3.279728542977952799, -3.411736077305369541, -0.2960517167220233503 ) ) ;
#9126=CARTESIAN_POINT ( 'NONE',  ( 4.900535883036028828, -2.496947748567499126, 3.359999999999999876 ) ) ;
#9130=CARTESIAN_POINT ( 'NONE',  ( 4.687928535947288644, -0.6479879772514620662, 4.216051716722023279 ) ) ;
#9135=CARTESIAN_POINT ( 'NONE',  ( -3.279728542977953687, 3.411736077305369541, 6.703948283277976650 ) ) ;
#9139=CARTESIAN_POINT ( 'NONE',  ( -0.7727076532861475444, -5.446173322633804048, 2.116051716722023190 ) ) ;
#9144=CARTESIAN_POINT ( 'NONE',  ( -4.215868657802586128, -2.148092372876348133, 9.939999999999997726 ) ) ;
#9149=CARTESIAN_POINT ( 'NONE',  ( -0.8323763977770610722, 4.658724279160015413, 6.176051716722023244 ) ) ;
#9160=CARTESIAN_POINT ( 'NONE',  ( 5.418398423912711870, 0.9480714621563913758, 4.076051716722022711 ) ) ;
#9162=CARTESIAN_POINT ( 'NONE',  ( -3.889087296526005044, -3.889087296526019255, 4.200000000000000178 ) ) ;
#9164=CARTESIAN_POINT ( 'NONE',  ( 3.889087296526005488, 3.889087296526018811, 5.599999999999998757 ) ) ;
#9177=CARTESIAN_POINT ( 'NONE',  ( 0.6479879772514793856, -4.687928535947285091, 5.583948283277975655 ) ) ;
#9183=CARTESIAN_POINT ( 'NONE',  ( -2.625446233515515537, -5.152728359536502545, 4.059999999999999609 ) ) ;
#9187=CARTESIAN_POINT ( 'NONE',  ( -2.064922774268895811, -4.258245684917318918, 10.65605171672202012 ) ) ;
#9189=CARTESIAN_POINT ( 'NONE',  ( 2.417848759854264618, -4.940838830814695548, 2.643948283277976596 ) ) ;
#9193=CARTESIAN_POINT ( 'NONE',  ( 2.625446233515515537, 5.152728359536502545, 13.85999999999999766 ) ) ;
#9198=CARTESIAN_POINT ( 'NONE',  ( 3.345732310141667387, -3.345732310141654064, 11.89999999999999858 ) ) ;
#9201=CARTESIAN_POINT ( 'NONE',  ( -3.119207202478379681, -3.244753828200550139, 13.59605171672202140 ) ) ;
#9210=CARTESIAN_POINT ( 'NONE',  ( -2.625446233515515981, -5.152728359536500768, 12.45999999999999552 ) ) ;
#9211=CARTESIAN_POINT ( 'NONE',  ( -0.8603895577212598011, -5.432285873273260179, 3.919999999999999929 ) ) ;
#9212=CARTESIAN_POINT ( 'NONE',  ( 5.711843387010018702, -0.9046671180729751738, 8.820000000000000284 ) ) ;
#9226=CARTESIAN_POINT ( 'NONE',  ( -3.969226411068985882, 2.122056237541205537, 9.363948283277975904 ) ) ;
#9235=CARTESIAN_POINT ( 'NONE',  ( -0.9046671180729962680, 5.711843387010016926, 13.57999999999999652 ) ) ;
#9240=CARTESIAN_POINT ( 'NONE',  ( -4.687928535947287756, 0.6479879772514611780, 14.01605171672202310 ) ) ;
#9243=CARTESIAN_POINT ( 'NONE',  ( 5.195105386651219348, 2.542276634908100075, 1.943948283277976419 ) ) ;
#9247=CARTESIAN_POINT ( 'NONE',  ( -0.9968613283357868893, 5.697241258616382531, 8.976051716722020402 ) ) ;
#9253=CARTESIAN_POINT ( 'NONE',  ( -4.215868657802586128, -2.148092372876348133, 7.139999999999998792 ) ) ;
#9254=CARTESIAN_POINT ( 'NONE',  ( -2.042957248827969252, 4.009529358847651714, 2.239999999999999769 ) ) ;
#9262=CARTESIAN_POINT ( 'NONE',  ( 0.9046671180729951578, -5.711843387010016926, 9.379999999999995453 ) ) ;
#9263=CARTESIAN_POINT ( 'NONE',  ( 2.496947748567516889, -4.900535883036019946, 12.03999999999999915 ) ) ;
#9264=CARTESIAN_POINT ( 'NONE',  ( -0.9046671180729963790, 5.711843387010016926, 5.179999999999999716 ) ) ;
#9276=CARTESIAN_POINT ( 'NONE',  ( -4.258245684917310925, -2.064922774268914019, 6.143948283277977040 ) ) ;
#9280=EDGE_CURVE ( 'NONE', #8250, #5138, #3621, .T. ) ;
#9281=CARTESIAN_POINT ( 'NONE',  ( 4.900535883036028828, -2.496947748567499126, 11.75999999999999979 ) ) ;
#9287=CARTESIAN_POINT ( 'NONE',  ( -4.173491630687863108, -2.231261971483782691, 13.73605171672202019 ) ) ;
#9291=CARTESIAN_POINT ( 'NONE',  ( 5.195105386651219348, 2.542276634908100075, -0.8560517167220232926 ) ) ;
#9300=CARTESIAN_POINT ( 'NONE',  ( -4.215868657802586128, -2.148092372876348133, 12.73999999999999844 ) ) ;
#9303=CARTESIAN_POINT ( 'NONE',  ( 4.673326407553653361, -0.7401821875142523544, 6.019999999999999574 ) ) ;
#9313=CARTESIAN_POINT ( 'NONE',  ( 3.889087296526005488, 3.889087296526018811, 11.19999999999999751 ) ) ;
#9314=CARTESIAN_POINT ( 'NONE',  ( -2.496947748567517333, 4.900535883036019058, 13.43999999999999950 ) ) ;
#9316=CARTESIAN_POINT ( 'NONE',  ( 5.432285873273257515, 0.8603895577212793411, 5.879999999999999893 ) ) ;
#9334=CARTESIAN_POINT ( 'NONE',  ( 1.963858260114715870, -4.049832306626327316, 5.443948283277975975 ) ) ;
#9346=CARTESIAN_POINT ( 'NONE',  ( 4.215868657802586128, 2.148092372876346801, 0.1400000000000000411 ) ) ;
#9348=CARTESIAN_POINT ( 'NONE',  ( -2.417848759854264618, 4.940838830814694660, 4.043948283277976508 ) ) ;
#9358=CARTESIAN_POINT ( 'NONE',  ( 3.181980515339458471, 3.181980515339470461, 13.99999999999999822 ) ) ;
#9360=CARTESIAN_POINT ( 'NONE',  ( -4.215868657802586128, -2.148092372876348133, 1.540000000000000036 ) ) ;
#9370=CARTESIAN_POINT ( 'NONE',  ( -4.155232146225753098, 4.023224611898306158, 11.49605171672201998 ) ) ;
#9371=CARTESIAN_POINT ( 'NONE',  ( 4.900535883036028828, -2.496947748567499126, 8.959999999999999076 ) ) ;
#9384=CARTESIAN_POINT ( 'NONE',  ( -0.6479879772514802738, 4.687928535947285091, 9.783948283277975833 ) ) ;
#9396=CARTESIAN_POINT ( 'NONE',  ( 4.009529358847659708, -2.042957248827953709, 0.5599999999999999423 ) ) ;
#9398=( GEOMETRIC_REPRESENTATION_CONTEXT ( 3 ) GLOBAL_UNCERTAINTY_ASSIGNED_CONTEXT ( ( #3888 ) ) GLOBAL_UNIT_ASSIGNED_CONTEXT ( ( #10391, #2111, #5543 ) ) REPRESENTATION_CONTEXT ( 'NONE', 'WORKASPACE' ) );
#9400=CARTESIAN_POINT ( 'NONE',  ( 3.244753828200538148, 3.119207202478391672, 10.20394828327797399 ) ) ;
#9403=ADVANCED_FACE ( 'NONE', ( #258 ), #3674, .T. ) ;
#9415=CARTESIAN_POINT ( 'NONE',  ( -0.7039550926810301812, -4.444597532678121965, 1.119999999999999885 ) ) ;
#9427=CARTESIAN_POINT ( 'NONE',  ( 3.826313983664925811, 3.951860609387098044, 9.396051716722022107 ) ) ;
#9434=( LENGTH_UNIT ( ) NAMED_UNIT ( * ) SI_UNIT ( .MILLI., .METRE. ) );
#9441=CARTESIAN_POINT ( 'NONE',  ( 5.697241258616385196, -0.9968613283357656840, 7.823948283277974980 ) ) ;
#9447=CARTESIAN_POINT ( 'NONE',  ( -4.900535883036028828, 2.496947748567499126, 13.15999999999999837 ) ) ;
#9452=CARTESIAN_POINT ( 'NONE',  ( 3.181980515339458471, 3.181980515339470461, 2.799999999999999378 ) ) ;
#9455=CARTESIAN_POINT ( 'NONE',  ( 5.697241258616385196, -0.9968613283357656840, 10.62394828327797569 ) ) ;
#9466=CARTESIAN_POINT ( 'NONE',  ( 0.7039550926810297371, 4.444597532678122853, 10.91999999999999993 ) ) ;
#9475=CARTESIAN_POINT ( 'NONE',  ( -4.155232146225753098, 4.023224611898306158, 5.896051716722023883 ) ) ;
#9479=ORIENTED_EDGE ( 'NONE', *, *, #984, .T. ) ;
#9493=CARTESIAN_POINT ( 'NONE',  ( 3.951860609387084722, 3.826313983664940022, 7.403948283277976827 ) ) ;
#9508=CARTESIAN_POINT ( 'NONE',  ( 0.7039550926810297371, 4.444597532678122853, 10.91999999999999993 ) ) ;
#9511=CARTESIAN_POINT ( 'NONE',  ( 3.951860609387084722, 3.826313983664940022, 10.20394828327797399 ) ) ;
#9525=CARTESIAN_POINT ( 'NONE',  ( -0.7401821875142701179, 4.673326407553649808, 10.77999999999999936 ) ) ;
#9531=FILL_AREA_STYLE_COLOUR ( '', #8980 ) ;
#9533=CARTESIAN_POINT ( 'NONE',  ( 3.826313983664925811, 3.951860609387098044, 6.596051716722022285 ) ) ;
#9538=CARTESIAN_POINT ( 'NONE',  ( -2.542276634908081423, -5.195105386651227342, 13.45605171672202260 ) ) ;
#9544=CARTESIAN_POINT ( 'NONE',  ( 3.889087296526005488, 3.889087296526018811, -3.866961113726609188E-17 ) ) ;
#9546=CARTESIAN_POINT ( 'NONE',  ( 4.023224611898322145, -4.155232146225737111, 2.503948283277976472 ) ) ;
#9561=CARTESIAN_POINT ( 'NONE',  ( 2.042957248827968808, -4.009529358847652603, 6.439999999999999503 ) ) ;
#9563=CARTESIAN_POINT ( 'NONE',  ( 5.446173322633801384, 0.7727076532861675284, 10.48394828327797512 ) ) ;
#9577=CARTESIAN_POINT ( 'NONE',  ( -2.042957248827969252, 4.009529358847651714, 7.839999999999999858 ) ) ;
#9586=CARTESIAN_POINT ( 'NONE',  ( -0.6162731882459178134, -4.458484982038665834, 7.716051716722023279 ) ) ;
#9590=CARTESIAN_POINT ( 'NONE',  ( -0.6162731882459178134, -4.458484982038665834, 2.116051716722023190 ) ) ;
#9600=CARTESIAN_POINT ( 'NONE',  ( 5.697241258616385196, -0.9968613283357656840, 5.023948283277976046 ) ) ;
#9613=CARTESIAN_POINT ( 'NONE',  ( -0.7401821875142701179, 4.673326407553649808, 10.77999999999999936 ) ) ;
#9618=CARTESIAN_POINT ( 'NONE',  ( 3.889087296526005488, 3.889087296526018811, -3.866961113726609188E-17 ) ) ;
#9631=CARTESIAN_POINT ( 'NONE',  ( 4.458484982038663169, 0.6162731882459350219, -0.7160517167220232793 ) ) ;
#9643=CARTESIAN_POINT ( 'NONE',  ( -3.119207202478379681, -3.244753828200550139, 2.396051716722022551 ) ) ;
#9651=CARTESIAN_POINT ( 'NONE',  ( -5.711843387010018702, 0.9046671180729746187, 7.419999999999998153 ) ) ;
#9653=CARTESIAN_POINT ( 'NONE',  ( 5.195105386651219348, 2.542276634908100075, 7.543948283277975619 ) ) ;
#9667=CARTESIAN_POINT ( 'NONE',  ( -0.7401821875142701179, 4.673326407553649808, 7.979999999999999538 ) ) ;
#9670=CARTESIAN_POINT ( 'NONE',  ( 5.195105386651219348, 2.542276634908100075, 7.543948283277975619 ) ) ;
#9676=CARTESIAN_POINT ( 'NONE',  ( 4.089228379062037178, -4.089228379062022967, 0.6999999999999997335 ) ) ;
#9688=CARTESIAN_POINT ( 'NONE',  ( 4.444597532678119300, 0.7039550926810472786, 8.679999999999997939 ) ) ;
#9698=CARTESIAN_POINT ( 'NONE',  ( -0.7039550926810301812, -4.444597532678121965, 1.119999999999999885 ) ) ;
#9701=CARTESIAN_POINT ( 'NONE',  ( 3.119207202478379681, 3.244753828200549695, 3.796051716722023350 ) ) ;
#9708=CARTESIAN_POINT ( 'NONE',  ( 5.711843387010018702, -0.9046671180729751738, 3.219999999999999751 ) ) ;
#9710=CARTESIAN_POINT ( 'NONE',  ( 5.446173322633801384, 0.7727076532861675284, 10.48394828327797512 ) ) ;
#9719=FACE_OUTER_BOUND ( 'NONE', #2360, .T. ) ;
#9720=CARTESIAN_POINT ( 'NONE',  ( -3.244753828200538148, -3.119207202478392116, 3.203948283277977094 ) ) ;
#9723=CARTESIAN_POINT ( 'NONE',  ( -4.089228379062038066, 4.089228379062021190, 7.699999999999998401 ) ) ;
#9727=CARTESIAN_POINT ( 'NONE',  ( 4.900535883036028828, -2.496947748567499126, 0.5599999999999999423 ) ) ;
#9737=CARTESIAN_POINT ( 'NONE',  ( 3.279728542977952799, -3.411736077305369541, 2.503948283277976472 ) ) ;
#9746=CARTESIAN_POINT ( 'NONE',  ( -3.181980515339458027, -3.181980515339470905, 4.200000000000000178 ) ) ;
#9752=CARTESIAN_POINT ( 'NONE',  ( -4.940838830814703542, 2.417848759854245078, 11.35605171672202296 ) ) ;
#9758=CARTESIAN_POINT ( 'NONE',  ( -4.089228379062038066, 4.089228379062021190, 2.099999999999999201 ) ) ;
#9759=CARTESIAN_POINT ( 'NONE',  ( 3.535533905932731980, 3.535533905932744414, 13.99999999999999822 ) ) ;
#9760=CARTESIAN_POINT ( 'NONE',  ( 3.951860609387084722, 3.826313983664940022, 13.00394828327797470 ) ) ;
#9773=CARTESIAN_POINT ( 'NONE',  ( 4.444597532678119300, 0.7039550926810472786, 11.47999999999999865 ) ) ;
#9776=CARTESIAN_POINT ( 'NONE',  ( 3.889087296526005488, 3.889087296526018811, 8.400000000000000355 ) ) ;
#9783=CARTESIAN_POINT ( 'NONE',  ( -2.122056237541221968, 3.969226411068977889, 3.236051716722023297 ) ) ;
#9785=CARTESIAN_POINT ( 'NONE',  ( 3.279728542977952799, -3.411736077305369541, 5.303948283277975406 ) ) ;
#9794=CARTESIAN_POINT ( 'NONE',  ( 4.444597532678119300, 0.7039550926810472786, 3.079999999999999627 ) ) ;
#9797=CARTESIAN_POINT ( 'NONE',  ( -0.6162731882459178134, -4.458484982038665834, 10.51605171672202133 ) ) ;
#9807=CARTESIAN_POINT ( 'NONE',  ( -5.711843387010018702, 0.9046671180729746187, 4.620000000000000107 ) ) ;
#9808=CARTESIAN_POINT ( 'NONE',  ( 4.089228379062037178, -4.089228379062022967, 6.299999999999999822 ) ) ;
#9809=CARTESIAN_POINT ( 'NONE',  ( 2.496947748567516889, -4.900535883036019946, 3.639999999999999680 ) ) ;
#9820=CARTESIAN_POINT ( 'NONE',  ( 4.658724279160018966, -0.8323763977770426425, -0.5760517167220230439 ) ) ;
#9825=CARTESIAN_POINT ( 'NONE',  ( 3.889087296526005488, 3.889087296526018811, 5.599999999999998757 ) ) ;
#9830=CARTESIAN_POINT ( 'NONE',  ( 5.711843387010019590, -0.9046671180729753958, 8.820000000000000284 ) ) ;
#9837=CARTESIAN_POINT ( 'NONE',  ( 4.049832306626335310, -1.963858260114701215, 7.156051716722023670 ) ) ;
#9840=CARTESIAN_POINT ( 'NONE',  ( 4.258245684917310037, 2.064922774268912686, 7.543948283277975619 ) ) ;
#9844=CARTESIAN_POINT ( 'NONE',  ( 2.576046737280769605, -4.860232935257343456, 4.636051716722022320 ) ) ;
#9851=CARTESIAN_POINT ( 'NONE',  ( -4.215868657802586128, -2.148092372876348133, 1.540000000000000036 ) ) ;
#9855=CARTESIAN_POINT ( 'NONE',  ( 2.122056237541221524, -3.969226411068978777, 10.23605171672202374 ) ) ;
#9864=CARTESIAN_POINT ( 'NONE',  ( -0.9046671180729963790, 5.711843387010016926, 2.379999999999999893 ) ) ;
#9865=CARTESIAN_POINT ( 'NONE',  ( -0.9480714621563718358, -5.418398423912716311, 11.32394828327797676 ) ) ;
#9876=CARTESIAN_POINT ( 'NONE',  ( 4.458484982038663169, 0.6162731882459350219, -0.7160517167220232793 ) ) ;
#9881=CARTESIAN_POINT ( 'NONE',  ( 5.432285873273257515, 0.8603895577212793411, 3.079999999999999627 ) ) ;
#9883=CARTESIAN_POINT ( 'NONE',  ( 5.711843387010019590, -0.9046671180729753958, 6.019999999999999574 ) ) ;
#9888=CARTESIAN_POINT ( 'NONE',  ( -4.155232146225753098, 4.023224611898306158, 14.29605171672202424 ) ) ;
#9891=CARTESIAN_POINT ( 'NONE',  ( -1.963858260114716980, 4.049832306626327316, 9.643948283277975264 ) ) ;
#9895=CARTESIAN_POINT ( 'NONE',  ( 5.418398423912711870, 0.9480714621563913758, 1.276051716722023333 ) ) ;
#9903=CARTESIAN_POINT ( 'NONE',  ( -3.119207202478379681, -3.244753828200550139, 7.996051716722022640 ) ) ;
#9906=PRODUCT_DEFINITION ( 'UNKNOWN', '', #7872, #3152 ) ;
#9912=CARTESIAN_POINT ( 'NONE',  ( -2.576046737280769605, 4.860232935257343456, 3.236051716722023297 ) ) ;
#9913=CARTESIAN_POINT ( 'NONE',  ( -2.625446233515515981, -5.152728359536500768, 6.859999999999999432 ) ) ;
#9915=CARTESIAN_POINT ( 'NONE',  ( 5.152728359536493663, 2.625446233515533745, 8.539999999999999147 ) ) ;
#9924=ORIENTED_EDGE ( 'NONE', *, *, #7662, .F. ) ;
#9929=CARTESIAN_POINT ( 'NONE',  ( -0.7916369971161423269, -4.430710083317576320, 0.1239482832779766203 ) ) ;
#9932=CARTESIAN_POINT ( 'NONE',  ( -5.152728359536494551, -2.625446233515535077, 1.540000000000000036 ) ) ;
#9935=CARTESIAN_POINT ( 'NONE',  ( 5.432285873273257515, 0.8603895577212793411, 11.47999999999999865 ) ) ;
#9942=CARTESIAN_POINT ( 'NONE',  ( -2.576046737280769605, 4.860232935257343456, 14.43605171672202125 ) ) ;
#9944=CARTESIAN_POINT ( 'NONE',  ( 3.244753828200538148, 3.119207202478391672, 1.803948283277976516 ) ) ;
#9947=CARTESIAN_POINT ( 'NONE',  ( -0.7727076532861475444, -5.446173322633804048, 4.916051716722023457 ) ) ;
#9952=CARTESIAN_POINT ( 'NONE',  ( 2.148092372876330369, 4.215868657802594122, 8.259999999999999787 ) ) ;
#9956=CARTESIAN_POINT ( 'NONE',  ( 0.6162731882459174804, 4.458484982038668498, 11.91605171672202346 ) ) ;
#9965=CARTESIAN_POINT ( 'NONE',  ( 3.826313983664925811, 3.951860609387098044, 3.796051716722023350 ) ) ;
#9966=CARTESIAN_POINT ( 'NONE',  ( 2.625446233515515537, 5.152728359536502545, 2.659999999999998366 ) ) ;
#9967=CARTESIAN_POINT ( 'NONE',  ( -2.625446233515515981, -5.152728359536500768, 12.45999999999999552 ) ) ;
#9978=CARTESIAN_POINT ( 'NONE',  ( -3.969226411068985882, 2.122056237541205537, 12.16394828327797661 ) ) ;
#9982=CARTESIAN_POINT ( 'NONE',  ( 0.9046671180729951578, -5.711843387010016926, 12.17999999999999439 ) ) ;
#9985=CARTESIAN_POINT ( 'NONE',  ( 4.900535883036028828, -2.496947748567499126, 11.75999999999999979 ) ) ;
#9990=CARTESIAN_POINT ( 'NONE',  ( -4.049832306626335310, 1.963858260114700327, 11.35605171672202296 ) ) ;
#9993=CARTESIAN_POINT ( 'NONE',  ( -4.458484982038663169, -0.6162731882459353550, 11.88394828327797548 ) ) ;
#9999=CARTESIAN_POINT ( 'NONE',  ( 4.155232146225751322, -4.023224611898307934, 4.496051716722022640 ) ) ;
#10004=CARTESIAN_POINT ( 'NONE',  ( -0.7039550926810301812, -4.444597532678121965, 9.519999999999999574 ) ) ;
#10005=CARTESIAN_POINT ( 'NONE',  ( -4.444597532678119300, -0.7039550926810477227, 1.679999999999999938 ) ) ;
#10019=CARTESIAN_POINT ( 'NONE',  ( 2.496947748567516889, -4.900535883036019946, 9.240000000000000213 ) ) ;
#10020=CARTESIAN_POINT ( 'NONE',  ( 4.089228379062037178, -4.089228379062022967, 0.6999999999999997335 ) ) ;
#10022=CARTESIAN_POINT ( 'NONE',  ( 0.9046671180729951578, -5.711843387010016926, 6.579999999999999183 ) ) ;
#10033=DIRECTION ( 'NONE',  ( -0.7071067811865465735, -0.7071067811865483499, 0.000000000000000000 ) ) ;
#10036=CARTESIAN_POINT ( 'NONE',  ( 3.244753828200538148, 3.119207202478391672, 10.20394828327797399 ) ) ;
#10042=CARTESIAN_POINT ( 'NONE',  ( 5.711843387010019590, -0.9046671180729753958, 3.219999999999999751 ) ) ;
#10046=CARTESIAN_POINT ( 'NONE',  ( -0.7401821875142701179, 4.673326407553649808, 2.379999999999999893 ) ) ;
#10048=CARTESIAN_POINT ( 'NONE',  ( 3.279728542977952799, -3.411736077305369541, 10.90394828327797327 ) ) ;
#10051=CARTESIAN_POINT ( 'NONE',  ( 3.826313983664925811, 3.951860609387098044, 3.796051716722023350 ) ) ;
#10056=CARTESIAN_POINT ( 'NONE',  ( 4.673326407553653361, -0.7401821875142525764, 8.820000000000000284 ) ) ;
#10059=CARTESIAN_POINT ( 'NONE',  ( 0.7039550926810297371, 4.444597532678122853, 5.319999999999999396 ) ) ;
#10067=CARTESIAN_POINT ( 'NONE',  ( -4.940838830814703542, 2.417848759854245078, 2.956051716722023492 ) ) ;
#10069=CARTESIAN_POINT ( 'NONE',  ( 4.089228379062037178, -4.089228379062022967, 9.099999999999999645 ) ) ;
#10070=CARTESIAN_POINT ( 'NONE',  ( 5.711843387010018702, -0.9046671180729751738, 11.61999999999999922 ) ) ;
#10083=CARTESIAN_POINT ( 'NONE',  ( 4.023224611898322145, -4.155232146225737111, -0.2960517167220233503 ) ) ;
#10087=CARTESIAN_POINT ( 'NONE',  ( -5.152728359536494551, -2.625446233515535077, 9.939999999999994174 ) ) ;
#10095=CARTESIAN_POINT ( 'NONE',  ( 4.430710083317573655, 0.7916369971161595354, 12.47605171672202218 ) ) ;
#10098=CARTESIAN_POINT ( 'NONE',  ( -2.417848759854264618, 4.940838830814694660, 1.243948283277976463 ) ) ;
#10107=CARTESIAN_POINT ( 'NONE',  ( -3.181980515339458027, -3.181980515339470905, 12.59999999999999787 ) ) ;
#10109=CARTESIAN_POINT ( 'NONE',  ( 4.215868657802586128, 2.148092372876346801, 2.939999999999999059 ) ) ;
#10120=CARTESIAN_POINT ( 'NONE',  ( 0.8603895577212593571, 5.432285873273261068, 10.91999999999999993 ) ) ;
#10121=CARTESIAN_POINT ( 'NONE',  ( -3.889087296526005044, -3.889087296526019255, 12.59999999999999787 ) ) ;
#10122=CARTESIAN_POINT ( 'NONE',  ( -0.8603895577212598011, -5.432285873273260179, 9.519999999999999574 ) ) ;
#10135=CARTESIAN_POINT ( 'NONE',  ( 0.6479879772514793856, -4.687928535947285091, 8.383948283277975477 ) ) ;
#10138=CARTESIAN_POINT ( 'NONE',  ( -2.496947748567517333, 4.900535883036019058, 10.63999999999999879 ) ) ;
#10145=CARTESIAN_POINT ( 'NONE',  ( 4.173491630687861331, 2.231261971483781359, 12.33605171672202339 ) ) ;
#10147=CARTESIAN_POINT ( 'NONE',  ( -4.860232935257354114, 2.576046737280751842, 3.763948283277976703 ) ) ;
#10157=CARTESIAN_POINT ( 'NONE',  ( -2.042957248827969252, 4.009529358847651714, 13.43999999999999950 ) ) ;
#10159=CARTESIAN_POINT ( 'NONE',  ( -4.430710083317573655, -0.7916369971161599794, 13.87605171672202253 ) ) ;
#10169=CARTESIAN_POINT ( 'NONE',  ( 0.9968613283357860011, -5.697241258616382531, 10.37605171672202253 ) ) ;
#10170=CARTESIAN_POINT ( 'NONE',  ( 4.900535883036028828, -2.496947748567499126, 11.75999999999999979 ) ) ;
#10187=CARTESIAN_POINT ( 'NONE',  ( -4.458484982038663169, -0.6162731882459353550, 6.283948283277974944 ) ) ;
#10194=CARTESIAN_POINT ( 'NONE',  ( -0.8603895577212598011, -5.432285873273260179, 12.31999999999999851 ) ) ;
#10195=CARTESIAN_POINT ( 'NONE',  ( 3.181980515339458471, 3.181980515339470461, 13.99999999999999822 ) ) ;
#10199=CARTESIAN_POINT ( 'NONE',  ( -4.687928535947287756, 0.6479879772514611780, 11.21605171672202417 ) ) ;
#10203=CARTESIAN_POINT ( 'NONE',  ( 0.9480714621563713917, 5.418398423912717199, 4.323948283277975868 ) ) ;
#10214=CARTESIAN_POINT ( 'NONE',  ( 0.8323763977770604061, -4.658724279160015413, 13.17605171672201969 ) ) ;
#10222=CARTESIAN_POINT ( 'NONE',  ( -4.940838830814703542, 2.417848759854245078, 8.556051716722022249 ) ) ;
#10236=CARTESIAN_POINT ( 'NONE',  ( 5.697241258616385196, -0.9968613283357656840, 2.223948283277975779 ) ) ;
#10247=CARTESIAN_POINT ( 'NONE',  ( -3.345732310141667831, 3.345732310141653620, 10.50000000000000000 ) ) ;
#10249=COLOUR_RGB ( '', 0.31764706, 0.68627451, 0.89019608) ;
#10250=CARTESIAN_POINT ( 'NONE',  ( -0.9480714621563718358, -5.418398423912716311, 5.723948283277976223 ) ) ;
#10265=CARTESIAN_POINT ( 'NONE',  ( -4.673326407553653361, 0.7401821875142517992, 13.01999999999999424 ) ) ;
#10273=( LENGTH_UNIT ( ) NAMED_UNIT ( * ) SI_UNIT ( .MILLI., .METRE. ) );
#10275=CARTESIAN_POINT ( 'NONE',  ( -2.542276634908081423, -5.195105386651227342, 10.65605171672202012 ) ) ;
#10287=CARTESIAN_POINT ( 'NONE',  ( -5.195105386651219348, -2.542276634908102295, 6.143948283277977040 ) ) ;
#10293=CARTESIAN_POINT ( 'NONE',  ( -2.496947748567517333, 4.900535883036019058, 13.43999999999999950 ) ) ;
#10299=CARTESIAN_POINT ( 'NONE',  ( -2.042957248827969252, 4.009529358847651714, 10.63999999999999879 ) ) ;
#10302=CARTESIAN_POINT ( 'NONE',  ( 5.195105386651219348, 2.542276634908100075, 4.743948283277974909 ) ) ;
#10312=CARTESIAN_POINT ( 'NONE',  ( 4.673326407553653361, -0.7401821875142523544, 8.820000000000000284 ) ) ;
#10320=CARTESIAN_POINT ( 'NONE',  ( -5.110351332421769754, -2.708615832122969191, 13.73605171672202019 ) ) ;
#10329=CARTESIAN_POINT ( 'NONE',  ( 5.726445515403654873, -0.8124729078101852187, 9.816051716722022036 ) ) ;
#10341=CARTESIAN_POINT ( 'NONE',  ( 0.8124729078102063129, -5.726445515403652209, 8.383948283277975477 ) ) ;
#10349=EDGE_LOOP ( 'NONE', ( #1291, #5274, #10, #7561 ) ) ;
#10358=CARTESIAN_POINT ( 'NONE',  ( 3.345732310141667387, -3.345732310141653620, 6.299999999999999822 ) ) ;
#10361=CARTESIAN_POINT ( 'NONE',  ( 2.417848759854264618, -4.940838830814695548, 8.243948283277976685 ) ) ;
#10374=CARTESIAN_POINT ( 'NONE',  ( -4.215868657802586128, -2.148092372876348133, 9.939999999999994174 ) ) ;
#10375=UNCERTAINTY_MEASURE_WITH_UNIT (LENGTH_MEASURE( 1.000000000000000082E-05 ), #9434, 'distance_accuracy_value', 'NONE');
#10383=CARTESIAN_POINT ( 'NONE',  ( -4.940838830814703542, 2.417848759854245078, 5.756051716722022427 ) ) ;
#10388=CARTESIAN_POINT ( 'NONE',  ( -3.826313983664925811, -3.951860609387098489, 10.79605171672202246 ) ) ;
#10389=PRODUCT_DEFINITION_SHAPE ( 'NONE', 'NONE',  #9906 ) ;
#10391=( LENGTH_UNIT ( ) NAMED_UNIT ( * ) SI_UNIT ( .MILLI., .METRE. ) );
#10400=CARTESIAN_POINT ( 'NONE',  ( 0.8124729078102063129, -5.726445515403652209, 5.583948283277975655 ) ) ;
#10412=CARTESIAN_POINT ( 'NONE',  ( 4.444597532678119300, 0.7039550926810472786, 8.679999999999997939 ) ) ;
#10414=CARTESIAN_POINT ( 'NONE',  ( -4.860232935257354114, 2.576046737280751842, 9.363948283277975904 ) ) ;
#10419=CARTESIAN_POINT ( 'NONE',  ( -5.432285873273256627, -0.8603895577212797852, 1.679999999999999938 ) ) ;
#10429=CARTESIAN_POINT ( 'NONE',  ( 2.148092372876330369, 4.215868657802593233, 13.85999999999999766 ) ) ;
#10444=CARTESIAN_POINT ( 'NONE',  ( -2.122056237541221968, 3.969226411068977889, 3.236051716722023297 ) ) ;
#10453=CARTESIAN_POINT ( 'NONE',  ( 2.625446233515515537, 5.152728359536502545, 2.659999999999998366 ) ) ;
#10455=CARTESIAN_POINT ( 'NONE',  ( -5.446173322633801384, -0.7727076532861678615, 3.483948283277976898 ) ) ;
#10468=CARTESIAN_POINT ( 'NONE',  ( -0.7039550926810301812, -4.444597532678121965, 6.719999999999999751 ) ) ;
#10474=CARTESIAN_POINT ( 'NONE',  ( -0.9480714621563718358, -5.418398423912716311, 8.523948283277976046 ) ) ;
#10486=CARTESIAN_POINT ( 'NONE',  ( -2.231261971483764484, -4.173491630687871101, 0.2639482832779765920 ) ) ;
#10497=CARTESIAN_POINT ( 'NONE',  ( -5.726445515403654873, 0.8124729078101847746, 11.21605171672202417 ) ) ;
ENDSEC;
END-ISO-10303-21;
